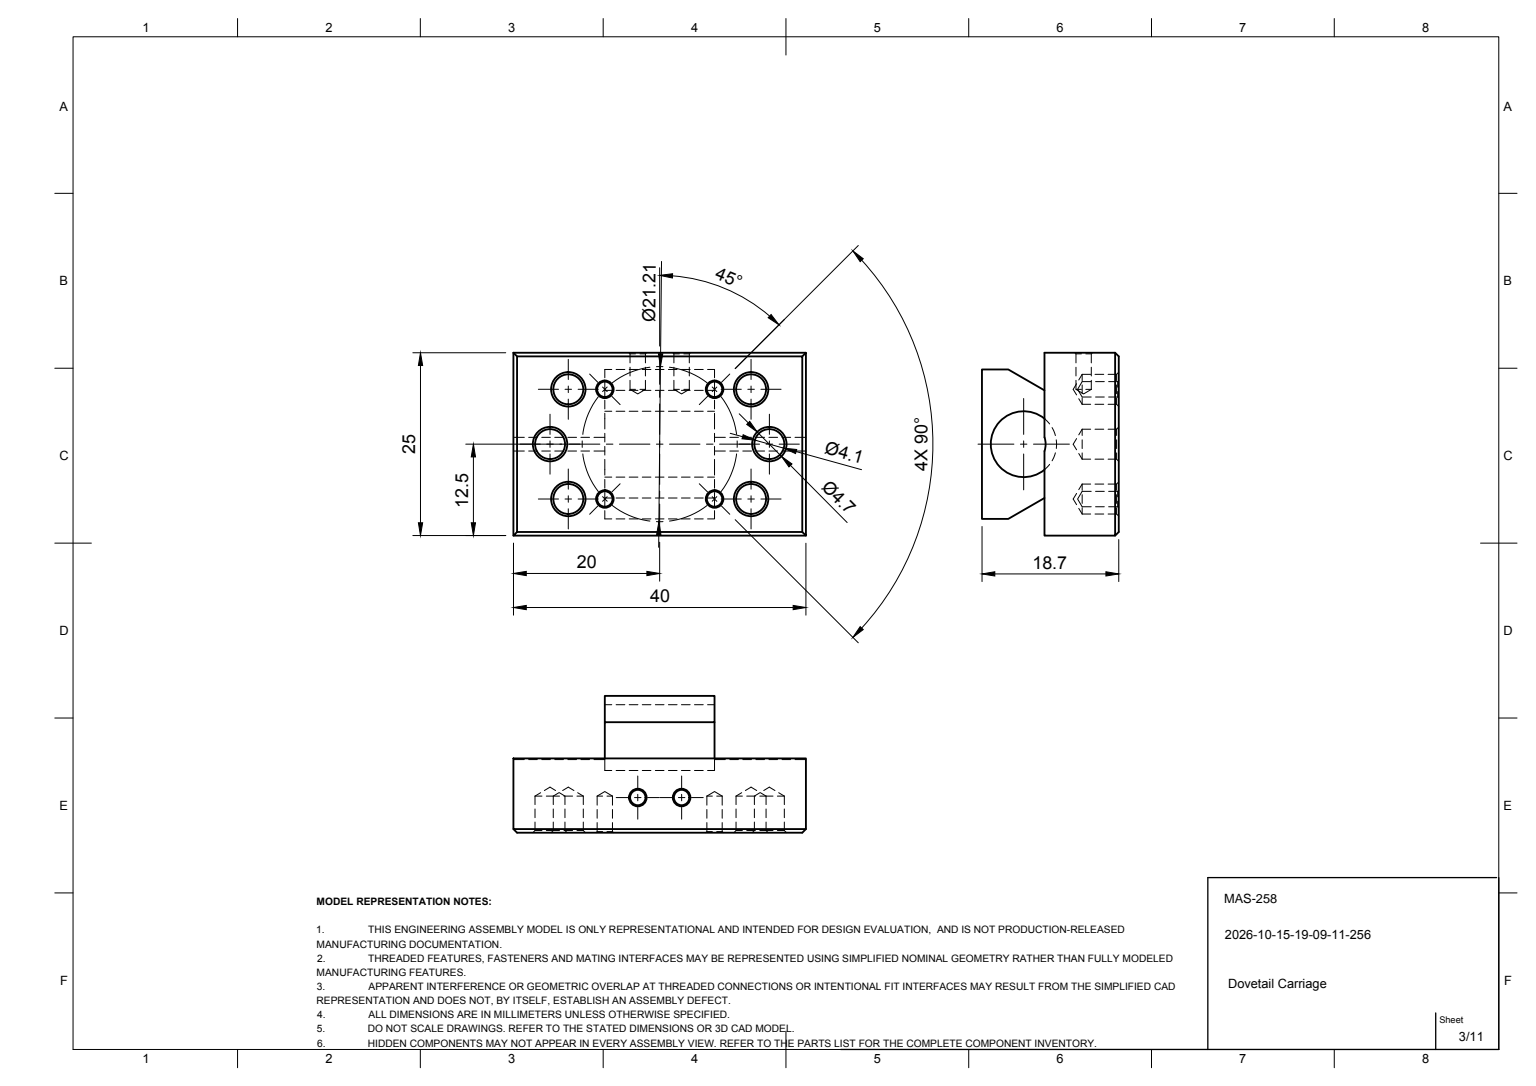
ISO-10303-21;
HEADER;
/* Generated by software containing ST-Developer
 * from STEP Tools, Inc. (www.steptools.com) 
 */

FILE_DESCRIPTION(
/* description */ (''),
/* implementation_level */ '2;1');

FILE_NAME(
/* name */ 'Dovetail Carriage.step',
/* time_stamp */ '2026-10-15T12:29:06-07:00',
/* author */ (''),
/* organization */ (''),
/* preprocessor_version */ 'ST-DEVELOPER v20.2',
/* originating_system */ 'Autodesk Translation Framework v15.15.0.0',
/* authorisation */ '');

FILE_SCHEMA (('AUTOMOTIVE_DESIGN { 1 0 10303 214 3 1 1 }'));
ENDSEC;

DATA;
#10=MECHANICAL_DESIGN_GEOMETRIC_PRESENTATION_REPRESENTATION('',(#1740),#135282);
#1714=SHAPE_REPRESENTATION_RELATIONSHIP('SRR','None',#135338,#1727);
#1727=ADVANCED_BREP_SHAPE_REPRESENTATION('',(#1753),#135270);
#1740=STYLED_ITEM('',(#135412),#1753);
#1753=MANIFOLD_SOLID_BREP('Body1',#32076);
#1769=CYLINDRICAL_SURFACE('',#32282,1.05);
#1770=CYLINDRICAL_SURFACE('',#32287,1.05);
#1771=CYLINDRICAL_SURFACE('',#32305,1.05);
#1772=CYLINDRICAL_SURFACE('',#32309,1.05);
#1773=CYLINDRICAL_SURFACE('',#32313,1.05);
#1774=CYLINDRICAL_SURFACE('',#32317,1.05);
#1775=CYLINDRICAL_SURFACE('',#32325,2.05);
#1776=CYLINDRICAL_SURFACE('',#32329,2.05);
#1777=CYLINDRICAL_SURFACE('',#32333,2.05);
#1778=CYLINDRICAL_SURFACE('',#32337,2.05);
#1779=CYLINDRICAL_SURFACE('',#32341,2.05);
#1780=CYLINDRICAL_SURFACE('',#32345,2.05);
#1781=CYLINDRICAL_SURFACE('',#32353,3.);
#1782=CYLINDRICAL_SURFACE('',#32358,3.);
#1783=CYLINDRICAL_SURFACE('',#32365,4.5);
#2020=FACE_BOUND('',#5136,.T.);
#2021=FACE_BOUND('',#5137,.T.);
#2022=FACE_BOUND('',#5145,.T.);
#2023=FACE_BOUND('',#5146,.T.);
#2024=FACE_BOUND('',#5147,.T.);
#2025=FACE_BOUND('',#5148,.T.);
#2026=FACE_BOUND('',#5149,.T.);
#2027=FACE_BOUND('',#5150,.T.);
#2028=FACE_BOUND('',#5151,.T.);
#2029=FACE_BOUND('',#5152,.T.);
#2030=FACE_BOUND('',#5153,.T.);
#2031=FACE_BOUND('',#5154,.T.);
#2250=PLANE('',#32280);
#2251=PLANE('',#32295);
#2252=PLANE('',#32356);
#2253=PLANE('',#32357);
#2254=PLANE('',#32361);
#2255=PLANE('',#32363);
#2256=PLANE('',#32370);
#2257=PLANE('',#32371);
#2258=PLANE('',#32372);
#2259=PLANE('',#32373);
#2260=PLANE('',#32374);
#2261=PLANE('',#32375);
#2262=PLANE('',#32376);
#2263=PLANE('',#32377);
#2264=PLANE('',#32378);
#2265=PLANE('',#32379);
#2266=PLANE('',#32380);
#2267=PLANE('',#32381);
#2268=PLANE('',#32382);
#2269=PLANE('',#32383);
#3376=FACE_OUTER_BOUND('',#5134,.T.);
#3377=FACE_OUTER_BOUND('',#5135,.T.);
#3378=FACE_OUTER_BOUND('',#5138,.T.);
#3379=FACE_OUTER_BOUND('',#5139,.T.);
#3380=FACE_OUTER_BOUND('',#5140,.T.);
#3381=FACE_OUTER_BOUND('',#5141,.T.);
#3382=FACE_OUTER_BOUND('',#5142,.T.);
#3383=FACE_OUTER_BOUND('',#5143,.T.);
#3384=FACE_OUTER_BOUND('',#5144,.T.);
#3385=FACE_OUTER_BOUND('',#5155,.T.);
#3386=FACE_OUTER_BOUND('',#5156,.T.);
#3387=FACE_OUTER_BOUND('',#5157,.T.);
#3388=FACE_OUTER_BOUND('',#5158,.T.);
#3389=FACE_OUTER_BOUND('',#5159,.T.);
#3390=FACE_OUTER_BOUND('',#5160,.T.);
#3391=FACE_OUTER_BOUND('',#5161,.T.);
#3392=FACE_OUTER_BOUND('',#5162,.T.);
#3393=FACE_OUTER_BOUND('',#5163,.T.);
#3394=FACE_OUTER_BOUND('',#5164,.T.);
#3395=FACE_OUTER_BOUND('',#5165,.T.);
#3396=FACE_OUTER_BOUND('',#5166,.T.);
#3397=FACE_OUTER_BOUND('',#5167,.T.);
#3398=FACE_OUTER_BOUND('',#5168,.T.);
#3399=FACE_OUTER_BOUND('',#5169,.T.);
#3400=FACE_OUTER_BOUND('',#5170,.T.);
#3401=FACE_OUTER_BOUND('',#5171,.T.);
#3402=FACE_OUTER_BOUND('',#5172,.T.);
#3403=FACE_OUTER_BOUND('',#5173,.T.);
#3404=FACE_OUTER_BOUND('',#5174,.T.);
#3405=FACE_OUTER_BOUND('',#5175,.T.);
#3406=FACE_OUTER_BOUND('',#5176,.T.);
#3407=FACE_OUTER_BOUND('',#5177,.T.);
#3408=FACE_OUTER_BOUND('',#5178,.T.);
#3409=FACE_OUTER_BOUND('',#5179,.T.);
#3410=FACE_OUTER_BOUND('',#5180,.T.);
#3411=FACE_OUTER_BOUND('',#5181,.T.);
#3412=FACE_OUTER_BOUND('',#5182,.T.);
#3413=FACE_OUTER_BOUND('',#5183,.T.);
#3414=FACE_OUTER_BOUND('',#5184,.T.);
#3415=FACE_OUTER_BOUND('',#5185,.T.);
#3416=FACE_OUTER_BOUND('',#5186,.T.);
#3417=FACE_OUTER_BOUND('',#5187,.T.);
#3418=FACE_OUTER_BOUND('',#5188,.T.);
#3419=FACE_OUTER_BOUND('',#5189,.T.);
#3420=FACE_OUTER_BOUND('',#5190,.T.);
#3421=FACE_OUTER_BOUND('',#5191,.T.);
#3422=FACE_OUTER_BOUND('',#5192,.T.);
#3423=FACE_OUTER_BOUND('',#5193,.T.);
#3424=FACE_OUTER_BOUND('',#5194,.T.);
#3425=FACE_OUTER_BOUND('',#5195,.T.);
#3426=FACE_OUTER_BOUND('',#5196,.T.);
#3427=FACE_OUTER_BOUND('',#5197,.T.);
#3428=FACE_OUTER_BOUND('',#5198,.T.);
#3429=FACE_OUTER_BOUND('',#5199,.T.);
#3430=FACE_OUTER_BOUND('',#5200,.T.);
#3431=FACE_OUTER_BOUND('',#5201,.T.);
#3432=FACE_OUTER_BOUND('',#5202,.T.);
#3433=FACE_OUTER_BOUND('',#5203,.T.);
#3434=FACE_OUTER_BOUND('',#5204,.T.);
#5134=EDGE_LOOP('',(#21120,#21121,#21122,#21123));
#5135=EDGE_LOOP('',(#21124,#21125,#21126,#21127));
#5136=EDGE_LOOP('',(#21128));
#5137=EDGE_LOOP('',(#21129));
#5138=EDGE_LOOP('',(#21130,#21131,#21132,#21133,#21134));
#5139=EDGE_LOOP('',(#21135,#21136,#21137,#21138));
#5140=EDGE_LOOP('',(#21139,#21140,#21141,#21142,#21143));
#5141=EDGE_LOOP('',(#21144,#21145,#21146,#21147));
#5142=EDGE_LOOP('',(#21148,#21149,#21150,#21151));
#5143=EDGE_LOOP('',(#21152,#21153,#21154,#21155));
#5144=EDGE_LOOP('',(#21156,#21157,#21158,#21159));
#5145=EDGE_LOOP('',(#21160));
#5146=EDGE_LOOP('',(#21161));
#5147=EDGE_LOOP('',(#21162));
#5148=EDGE_LOOP('',(#21163));
#5149=EDGE_LOOP('',(#21164));
#5150=EDGE_LOOP('',(#21165));
#5151=EDGE_LOOP('',(#21166));
#5152=EDGE_LOOP('',(#21167));
#5153=EDGE_LOOP('',(#21168));
#5154=EDGE_LOOP('',(#21169));
#5155=EDGE_LOOP('',(#21170,#21171,#21172,#21173));
#5156=EDGE_LOOP('',(#21174,#21175,#21176,#21177));
#5157=EDGE_LOOP('',(#21178,#21179,#21180,#21181));
#5158=EDGE_LOOP('',(#21182,#21183,#21184,#21185));
#5159=EDGE_LOOP('',(#21186,#21187,#21188,#21189));
#5160=EDGE_LOOP('',(#21190,#21191,#21192,#21193));
#5161=EDGE_LOOP('',(#21194,#21195,#21196,#21197));
#5162=EDGE_LOOP('',(#21198,#21199,#21200));
#5163=EDGE_LOOP('',(#21201,#21202,#21203));
#5164=EDGE_LOOP('',(#21204,#21205,#21206));
#5165=EDGE_LOOP('',(#21207,#21208,#21209));
#5166=EDGE_LOOP('',(#21210,#21211,#21212,#21213));
#5167=EDGE_LOOP('',(#21214,#21215,#21216,#21217));
#5168=EDGE_LOOP('',(#21218,#21219,#21220,#21221));
#5169=EDGE_LOOP('',(#21222,#21223,#21224,#21225));
#5170=EDGE_LOOP('',(#21226,#21227,#21228,#21229));
#5171=EDGE_LOOP('',(#21230,#21231,#21232,#21233));
#5172=EDGE_LOOP('',(#21234,#21235,#21236,#21237));
#5173=EDGE_LOOP('',(#21238,#21239,#21240,#21241));
#5174=EDGE_LOOP('',(#21242,#21243,#21244,#21245));
#5175=EDGE_LOOP('',(#21246,#21247,#21248,#21249));
#5176=EDGE_LOOP('',(#21250,#21251,#21252,#21253));
#5177=EDGE_LOOP('',(#21254,#21255,#21256,#21257));
#5178=EDGE_LOOP('',(#21258,#21259,#21260));
#5179=EDGE_LOOP('',(#21261,#21262,#21263));
#5180=EDGE_LOOP('',(#21264,#21265,#21266));
#5181=EDGE_LOOP('',(#21267,#21268,#21269));
#5182=EDGE_LOOP('',(#21270,#21271,#21272));
#5183=EDGE_LOOP('',(#21273,#21274,#21275));
#5184=EDGE_LOOP('',(#21276,#21277,#21278,#21279));
#5185=EDGE_LOOP('',(#21280,#21281,#21282,#21283,#21284,#21285));
#5186=EDGE_LOOP('',(#21286,#21287,#21288,#21289,#21290,#21291,#21292,#21293,
#21294,#21295));
#5187=EDGE_LOOP('',(#21296,#21297,#21298,#21299));
#5188=EDGE_LOOP('',(#21300,#21301,#21302,#21303));
#5189=EDGE_LOOP('',(#21304,#21305,#21306,#21307));
#5190=EDGE_LOOP('',(#21308,#21309,#21310,#21311,#21312,#21313,#21314,#21315));
#5191=EDGE_LOOP('',(#21316,#21317,#21318,#21319));
#5192=EDGE_LOOP('',(#21320,#21321,#21322,#21323));
#5193=EDGE_LOOP('',(#21324,#21325,#21326,#21327));
#5194=EDGE_LOOP('',(#21328,#21329,#21330,#21331));
#5195=EDGE_LOOP('',(#21332,#21333,#21334,#21335,#21336,#21337));
#5196=EDGE_LOOP('',(#21338,#21339,#21340,#21341,#21342,#21343,#21344,#21345,
#21346));
#5197=EDGE_LOOP('',(#21347,#21348,#21349,#21350));
#5198=EDGE_LOOP('',(#21351,#21352,#21353,#21354));
#5199=EDGE_LOOP('',(#21355,#21356,#21357,#21358));
#5200=EDGE_LOOP('',(#21359,#21360,#21361,#21362));
#5201=EDGE_LOOP('',(#21363,#21364,#21365,#21366));
#5202=EDGE_LOOP('',(#21367,#21368,#21369,#21370,#21371,#21372,#21373,#21374,
#21375));
#5203=EDGE_LOOP('',(#21376,#21377,#21378,#21379));
#5204=EDGE_LOOP('',(#21380,#21381,#21382,#21383,#21384,#21385,#21386,#21387,
#21388,#21389));
#7130=LINE('',#41202,#9967);
#7131=LINE('',#41207,#9968);
#7132=LINE('',#41209,#9969);
#7133=LINE('',#41211,#9970);
#7134=LINE('',#41212,#9971);
#7135=LINE('',#41217,#9972);
#7136=LINE('',#41224,#9973);
#7137=LINE('',#41227,#9974);
#7138=LINE('',#41233,#9975);
#7139=LINE('',#41236,#9976);
#7140=LINE('',#41241,#9977);
#7141=LINE('',#41246,#9978);
#7142=LINE('',#41248,#9979);
#7143=LINE('',#41250,#9980);
#7144=LINE('',#41251,#9981);
#7145=LINE('',#41272,#9982);
#7146=LINE('',#41277,#9983);
#7147=LINE('',#41280,#9984);
#7148=LINE('',#41285,#9985);
#7149=LINE('',#41288,#9986);
#7150=LINE('',#41293,#9987);
#7151=LINE('',#41296,#9988);
#7152=LINE('',#41300,#9989);
#7153=LINE('',#41303,#9990);
#7154=LINE('',#41306,#9991);
#7155=LINE('',#41309,#9992);
#7156=LINE('',#41313,#9993);
#7157=LINE('',#41316,#9994);
#7158=LINE('',#41321,#9995);
#7159=LINE('',#41324,#9996);
#7160=LINE('',#41329,#9997);
#7161=LINE('',#41332,#9998);
#7162=LINE('',#41337,#9999);
#7163=LINE('',#41340,#10000);
#7164=LINE('',#41345,#10001);
#7165=LINE('',#41348,#10002);
#7166=LINE('',#41353,#10003);
#7167=LINE('',#41356,#10004);
#7168=LINE('',#41360,#10005);
#7169=LINE('',#41363,#10006);
#7170=LINE('',#41366,#10007);
#7171=LINE('',#41369,#10008);
#7172=LINE('',#41372,#10009);
#7173=LINE('',#41375,#10010);
#7174=LINE('',#41379,#10011);
#7175=LINE('',#41383,#10012);
#7176=LINE('',#41387,#10013);
#7177=LINE('',#41389,#10014);
#7178=LINE('',#41390,#10015);
#7179=LINE('',#41391,#10016);
#7180=LINE('',#41394,#10017);
#7181=LINE('',#41396,#10018);
#7182=LINE('',#41398,#10019);
#7183=LINE('',#41400,#10020);
#7184=LINE('',#41402,#10021);
#7185=LINE('',#41404,#10022);
#7186=LINE('',#41406,#10023);
#7187=LINE('',#41407,#10024);
#7188=LINE('',#41411,#10025);
#7189=LINE('',#41417,#10026);
#7190=LINE('',#41420,#10027);
#7191=LINE('',#41427,#10028);
#7192=LINE('',#41432,#10029);
#7193=LINE('',#41433,#10030);
#7194=LINE('',#41434,#10031);
#7195=LINE('',#41436,#10032);
#7196=LINE('',#41437,#10033);
#7197=LINE('',#41439,#10034);
#7198=LINE('',#41442,#10035);
#7199=LINE('',#41443,#10036);
#7200=LINE('',#41446,#10037);
#7201=LINE('',#41448,#10038);
#7202=LINE('',#41450,#10039);
#7203=LINE('',#41452,#10040);
#7204=LINE('',#41454,#10041);
#7205=LINE('',#41455,#10042);
#7206=LINE('',#41458,#10043);
#7207=LINE('',#41459,#10044);
#7208=LINE('',#41462,#10045);
#7209=LINE('',#41463,#10046);
#7210=LINE('',#41466,#10047);
#7211=LINE('',#41467,#10048);
#7212=LINE('',#41470,#10049);
#7213=LINE('',#41471,#10050);
#7214=LINE('',#41474,#10051);
#7215=LINE('',#41475,#10052);
#7216=LINE('',#41477,#10053);
#9967=VECTOR('',#34378,1.125);
#9968=VECTOR('',#34383,10.);
#9969=VECTOR('',#34384,10.);
#9970=VECTOR('',#34385,10.);
#9971=VECTOR('',#34386,10.);
#9972=VECTOR('',#34391,1.05);
#9973=VECTOR('',#34400,1.125);
#9974=VECTOR('',#34403,1.05);
#9975=VECTOR('',#34410,0.524999999999993);
#9976=VECTOR('',#34413,0.524999999999993);
#9977=VECTOR('',#34418,1.125);
#9978=VECTOR('',#34423,10.);
#9979=VECTOR('',#34424,10.);
#9980=VECTOR('',#34425,10.);
#9981=VECTOR('',#34426,10.);
#9982=VECTOR('',#34447,1.05);
#9983=VECTOR('',#34454,1.125);
#9984=VECTOR('',#34457,1.05);
#9985=VECTOR('',#34464,1.125);
#9986=VECTOR('',#34467,1.05);
#9987=VECTOR('',#34474,1.125);
#9988=VECTOR('',#34477,1.05);
#9989=VECTOR('',#34482,0.525);
#9990=VECTOR('',#34485,0.525);
#9991=VECTOR('',#34488,0.525);
#9992=VECTOR('',#34491,0.525);
#9993=VECTOR('',#34496,2.2);
#9994=VECTOR('',#34499,2.05);
#9995=VECTOR('',#34506,2.2);
#9996=VECTOR('',#34509,2.05);
#9997=VECTOR('',#34516,2.2);
#9998=VECTOR('',#34519,2.05);
#9999=VECTOR('',#34526,2.2);
#10000=VECTOR('',#34529,2.05);
#10001=VECTOR('',#34536,2.2);
#10002=VECTOR('',#34539,2.05);
#10003=VECTOR('',#34546,2.2);
#10004=VECTOR('',#34549,2.05);
#10005=VECTOR('',#34554,1.025);
#10006=VECTOR('',#34557,1.025);
#10007=VECTOR('',#34560,1.025);
#10008=VECTOR('',#34563,1.025);
#10009=VECTOR('',#34566,1.025);
#10010=VECTOR('',#34569,1.025);
#10011=VECTOR('',#34572,10.);
#10012=VECTOR('',#34575,10.);
#10013=VECTOR('',#34580,10.);
#10014=VECTOR('',#34581,10.);
#10015=VECTOR('',#34582,10.);
#10016=VECTOR('',#34583,10.);
#10017=VECTOR('',#34586,10.);
#10018=VECTOR('',#34587,10.);
#10019=VECTOR('',#34588,10.);
#10020=VECTOR('',#34589,10.);
#10021=VECTOR('',#34590,10.);
#10022=VECTOR('',#34591,10.);
#10023=VECTOR('',#34592,10.);
#10024=VECTOR('',#34593,10.);
#10025=VECTOR('',#34596,10.);
#10026=VECTOR('',#34605,10.);
#10027=VECTOR('',#34608,10.);
#10028=VECTOR('',#34617,4.5);
#10029=VECTOR('',#34624,10.);
#10030=VECTOR('',#34625,10.);
#10031=VECTOR('',#34626,10.);
#10032=VECTOR('',#34629,10.);
#10033=VECTOR('',#34630,10.);
#10034=VECTOR('',#34633,10.);
#10035=VECTOR('',#34638,10.);
#10036=VECTOR('',#34639,10.);
#10037=VECTOR('',#34642,10.);
#10038=VECTOR('',#34643,10.);
#10039=VECTOR('',#34644,10.);
#10040=VECTOR('',#34645,10.);
#10041=VECTOR('',#34646,10.);
#10042=VECTOR('',#34647,10.);
#10043=VECTOR('',#34650,10.);
#10044=VECTOR('',#34651,10.);
#10045=VECTOR('',#34654,10.);
#10046=VECTOR('',#34655,10.);
#10047=VECTOR('',#34658,10.);
#10048=VECTOR('',#34659,10.);
#10049=VECTOR('',#34662,10.);
#10050=VECTOR('',#34663,10.);
#10051=VECTOR('',#34666,10.);
#10052=VECTOR('',#34667,10.);
#10053=VECTOR('',#34670,10.);
#12756=CIRCLE('',#32278,1.05);
#12757=CIRCLE('',#32279,1.2);
#12758=CIRCLE('',#32281,1.2);
#12759=CIRCLE('',#32283,1.05);
#12760=CIRCLE('',#32284,1.05);
#12761=CIRCLE('',#32286,1.05);
#12762=CIRCLE('',#32288,1.05);
#12763=CIRCLE('',#32289,1.05);
#12764=CIRCLE('',#32293,1.05);
#12765=CIRCLE('',#32294,1.2);
#12766=CIRCLE('',#32296,1.2);
#12767=CIRCLE('',#32297,1.2);
#12768=CIRCLE('',#32298,2.35);
#12769=CIRCLE('',#32299,2.35);
#12770=CIRCLE('',#32300,2.35);
#12771=CIRCLE('',#32301,2.35);
#12772=CIRCLE('',#32302,2.35);
#12773=CIRCLE('',#32303,2.35);
#12774=CIRCLE('',#32304,1.2);
#12775=CIRCLE('',#32306,1.05);
#12776=CIRCLE('',#32308,1.05);
#12777=CIRCLE('',#32310,1.05);
#12778=CIRCLE('',#32312,1.05);
#12779=CIRCLE('',#32314,1.05);
#12780=CIRCLE('',#32316,1.05);
#12781=CIRCLE('',#32318,1.05);
#12782=CIRCLE('',#32324,2.05);
#12783=CIRCLE('',#32326,2.05);
#12784=CIRCLE('',#32328,2.05);
#12785=CIRCLE('',#32330,2.05);
#12786=CIRCLE('',#32332,2.05);
#12787=CIRCLE('',#32334,2.05);
#12788=CIRCLE('',#32336,2.05);
#12789=CIRCLE('',#32338,2.05);
#12790=CIRCLE('',#32340,2.05);
#12791=CIRCLE('',#32342,2.05);
#12792=CIRCLE('',#32344,2.05);
#12793=CIRCLE('',#32346,2.05);
#12794=CIRCLE('',#32354,3.);
#12795=CIRCLE('',#32355,3.);
#12796=CIRCLE('',#32359,3.);
#12797=CIRCLE('',#32360,3.);
#12798=CIRCLE('',#32362,4.5);
#12799=CIRCLE('',#32364,4.5);
#12800=CIRCLE('',#32366,4.5);
#12801=CIRCLE('',#32367,4.5);
#12802=CIRCLE('',#32368,4.5);
#12803=CIRCLE('',#32369,4.5);
#13292=VERTEX_POINT('',#41199);
#13293=VERTEX_POINT('',#41201);
#13294=VERTEX_POINT('',#41205);
#13295=VERTEX_POINT('',#41206);
#13296=VERTEX_POINT('',#41208);
#13297=VERTEX_POINT('',#41210);
#13298=VERTEX_POINT('',#41213);
#13299=VERTEX_POINT('',#41216);
#13300=VERTEX_POINT('',#41218);
#13301=VERTEX_POINT('',#41222);
#13302=VERTEX_POINT('',#41226);
#13303=VERTEX_POINT('',#41228);
#13304=VERTEX_POINT('',#41232);
#13305=VERTEX_POINT('',#41235);
#13306=VERTEX_POINT('',#41238);
#13307=VERTEX_POINT('',#41240);
#13308=VERTEX_POINT('',#41244);
#13309=VERTEX_POINT('',#41245);
#13310=VERTEX_POINT('',#41247);
#13311=VERTEX_POINT('',#41249);
#13312=VERTEX_POINT('',#41252);
#13313=VERTEX_POINT('',#41254);
#13314=VERTEX_POINT('',#41256);
#13315=VERTEX_POINT('',#41258);
#13316=VERTEX_POINT('',#41260);
#13317=VERTEX_POINT('',#41262);
#13318=VERTEX_POINT('',#41264);
#13319=VERTEX_POINT('',#41266);
#13320=VERTEX_POINT('',#41268);
#13321=VERTEX_POINT('',#41271);
#13322=VERTEX_POINT('',#41275);
#13323=VERTEX_POINT('',#41279);
#13324=VERTEX_POINT('',#41283);
#13325=VERTEX_POINT('',#41287);
#13326=VERTEX_POINT('',#41291);
#13327=VERTEX_POINT('',#41295);
#13328=VERTEX_POINT('',#41299);
#13329=VERTEX_POINT('',#41302);
#13330=VERTEX_POINT('',#41305);
#13331=VERTEX_POINT('',#41308);
#13332=VERTEX_POINT('',#41311);
#13333=VERTEX_POINT('',#41315);
#13334=VERTEX_POINT('',#41319);
#13335=VERTEX_POINT('',#41323);
#13336=VERTEX_POINT('',#41327);
#13337=VERTEX_POINT('',#41331);
#13338=VERTEX_POINT('',#41335);
#13339=VERTEX_POINT('',#41339);
#13340=VERTEX_POINT('',#41343);
#13341=VERTEX_POINT('',#41347);
#13342=VERTEX_POINT('',#41351);
#13343=VERTEX_POINT('',#41355);
#13344=VERTEX_POINT('',#41359);
#13345=VERTEX_POINT('',#41362);
#13346=VERTEX_POINT('',#41365);
#13347=VERTEX_POINT('',#41368);
#13348=VERTEX_POINT('',#41371);
#13349=VERTEX_POINT('',#41374);
#13350=VERTEX_POINT('',#41377);
#13351=VERTEX_POINT('',#41378);
#13352=VERTEX_POINT('',#41380);
#13353=VERTEX_POINT('',#41382);
#13354=VERTEX_POINT('',#41386);
#13355=VERTEX_POINT('',#41388);
#13356=VERTEX_POINT('',#41393);
#13357=VERTEX_POINT('',#41395);
#13358=VERTEX_POINT('',#41397);
#13359=VERTEX_POINT('',#41399);
#13360=VERTEX_POINT('',#41401);
#13361=VERTEX_POINT('',#41403);
#13362=VERTEX_POINT('',#41405);
#13363=VERTEX_POINT('',#41409);
#13364=VERTEX_POINT('',#41410);
#13365=VERTEX_POINT('',#41415);
#13366=VERTEX_POINT('',#41419);
#13367=VERTEX_POINT('',#41423);
#13368=VERTEX_POINT('',#41426);
#13369=VERTEX_POINT('',#41431);
#13370=VERTEX_POINT('',#41445);
#13371=VERTEX_POINT('',#41447);
#13372=VERTEX_POINT('',#41449);
#13373=VERTEX_POINT('',#41451);
#13374=VERTEX_POINT('',#41453);
#13375=VERTEX_POINT('',#41457);
#13376=VERTEX_POINT('',#41461);
#13377=VERTEX_POINT('',#41465);
#13378=VERTEX_POINT('',#41469);
#13379=VERTEX_POINT('',#41473);
#16411=EDGE_CURVE('',#13292,#13292,#12756,.T.);
#16412=EDGE_CURVE('',#13292,#13293,#7130,.T.);
#16413=EDGE_CURVE('',#13293,#13293,#12757,.T.);
#16414=EDGE_CURVE('',#13294,#13295,#7131,.T.);
#16415=EDGE_CURVE('',#13296,#13294,#7132,.T.);
#16416=EDGE_CURVE('',#13296,#13297,#7133,.T.);
#16417=EDGE_CURVE('',#13295,#13297,#7134,.T.);
#16418=EDGE_CURVE('',#13298,#13298,#12758,.T.);
#16419=EDGE_CURVE('',#13292,#13299,#7135,.T.);
#16420=EDGE_CURVE('',#13299,#13300,#12759,.T.);
#16421=EDGE_CURVE('',#13300,#13299,#12760,.T.);
#16422=EDGE_CURVE('',#13301,#13301,#12761,.T.);
#16423=EDGE_CURVE('',#13301,#13298,#7136,.T.);
#16424=EDGE_CURVE('',#13301,#13302,#7137,.T.);
#16425=EDGE_CURVE('',#13302,#13303,#12762,.T.);
#16426=EDGE_CURVE('',#13303,#13302,#12763,.T.);
#16427=EDGE_CURVE('',#13304,#13300,#7138,.T.);
#16428=EDGE_CURVE('',#13305,#13303,#7139,.T.);
#16429=EDGE_CURVE('',#13306,#13306,#12764,.T.);
#16430=EDGE_CURVE('',#13306,#13307,#7140,.T.);
#16431=EDGE_CURVE('',#13307,#13307,#12765,.T.);
#16432=EDGE_CURVE('',#13308,#13309,#7141,.T.);
#16433=EDGE_CURVE('',#13310,#13308,#7142,.T.);
#16434=EDGE_CURVE('',#13311,#13310,#7143,.T.);
#16435=EDGE_CURVE('',#13309,#13311,#7144,.T.);
#16436=EDGE_CURVE('',#13312,#13312,#12766,.T.);
#16437=EDGE_CURVE('',#13313,#13313,#12767,.T.);
#16438=EDGE_CURVE('',#13314,#13314,#12768,.T.);
#16439=EDGE_CURVE('',#13315,#13315,#12769,.T.);
#16440=EDGE_CURVE('',#13316,#13316,#12770,.T.);
#16441=EDGE_CURVE('',#13317,#13317,#12771,.T.);
#16442=EDGE_CURVE('',#13318,#13318,#12772,.T.);
#16443=EDGE_CURVE('',#13319,#13319,#12773,.T.);
#16444=EDGE_CURVE('',#13320,#13320,#12774,.T.);
#16445=EDGE_CURVE('',#13306,#13321,#7145,.T.);
#16446=EDGE_CURVE('',#13321,#13321,#12775,.T.);
#16447=EDGE_CURVE('',#13322,#13322,#12776,.T.);
#16448=EDGE_CURVE('',#13322,#13312,#7146,.T.);
#16449=EDGE_CURVE('',#13322,#13323,#7147,.T.);
#16450=EDGE_CURVE('',#13323,#13323,#12777,.T.);
#16451=EDGE_CURVE('',#13324,#13324,#12778,.T.);
#16452=EDGE_CURVE('',#13324,#13320,#7148,.T.);
#16453=EDGE_CURVE('',#13324,#13325,#7149,.T.);
#16454=EDGE_CURVE('',#13325,#13325,#12779,.T.);
#16455=EDGE_CURVE('',#13326,#13326,#12780,.T.);
#16456=EDGE_CURVE('',#13326,#13313,#7150,.T.);
#16457=EDGE_CURVE('',#13326,#13327,#7151,.T.);
#16458=EDGE_CURVE('',#13327,#13327,#12781,.T.);
#16459=EDGE_CURVE('',#13328,#13321,#7152,.T.);
#16460=EDGE_CURVE('',#13329,#13327,#7153,.T.);
#16461=EDGE_CURVE('',#13330,#13325,#7154,.T.);
#16462=EDGE_CURVE('',#13331,#13323,#7155,.T.);
#16463=EDGE_CURVE('',#13332,#13332,#12782,.T.);
#16464=EDGE_CURVE('',#13332,#13314,#7156,.T.);
#16465=EDGE_CURVE('',#13332,#13333,#7157,.T.);
#16466=EDGE_CURVE('',#13333,#13333,#12783,.T.);
#16467=EDGE_CURVE('',#13334,#13334,#12784,.T.);
#16468=EDGE_CURVE('',#13334,#13319,#7158,.T.);
#16469=EDGE_CURVE('',#13334,#13335,#7159,.T.);
#16470=EDGE_CURVE('',#13335,#13335,#12785,.T.);
#16471=EDGE_CURVE('',#13336,#13336,#12786,.T.);
#16472=EDGE_CURVE('',#13336,#13315,#7160,.T.);
#16473=EDGE_CURVE('',#13336,#13337,#7161,.T.);
#16474=EDGE_CURVE('',#13337,#13337,#12787,.T.);
#16475=EDGE_CURVE('',#13338,#13338,#12788,.T.);
#16476=EDGE_CURVE('',#13338,#13318,#7162,.T.);
#16477=EDGE_CURVE('',#13338,#13339,#7163,.T.);
#16478=EDGE_CURVE('',#13339,#13339,#12789,.T.);
#16479=EDGE_CURVE('',#13340,#13340,#12790,.T.);
#16480=EDGE_CURVE('',#13340,#13316,#7164,.T.);
#16481=EDGE_CURVE('',#13340,#13341,#7165,.T.);
#16482=EDGE_CURVE('',#13341,#13341,#12791,.T.);
#16483=EDGE_CURVE('',#13342,#13342,#12792,.T.);
#16484=EDGE_CURVE('',#13342,#13317,#7166,.T.);
#16485=EDGE_CURVE('',#13342,#13343,#7167,.T.);
#16486=EDGE_CURVE('',#13343,#13343,#12793,.T.);
#16487=EDGE_CURVE('',#13344,#13333,#7168,.T.);
#16488=EDGE_CURVE('',#13345,#13343,#7169,.T.);
#16489=EDGE_CURVE('',#13346,#13335,#7170,.T.);
#16490=EDGE_CURVE('',#13347,#13337,#7171,.T.);
#16491=EDGE_CURVE('',#13348,#13339,#7172,.T.);
#16492=EDGE_CURVE('',#13349,#13341,#7173,.T.);
#16493=EDGE_CURVE('',#13350,#13351,#7174,.T.);
#16494=EDGE_CURVE('',#13352,#13350,#12794,.T.);
#16495=EDGE_CURVE('',#13353,#13352,#7175,.T.);
#16496=EDGE_CURVE('',#13351,#13353,#12795,.T.);
#16497=EDGE_CURVE('',#13353,#13354,#7176,.T.);
#16498=EDGE_CURVE('',#13354,#13355,#7177,.T.);
#16499=EDGE_CURVE('',#13295,#13355,#7178,.T.);
#16500=EDGE_CURVE('',#13297,#13351,#7179,.T.);
#16501=EDGE_CURVE('',#13352,#13356,#7180,.T.);
#16502=EDGE_CURVE('',#13356,#13357,#7181,.T.);
#16503=EDGE_CURVE('',#13357,#13358,#7182,.T.);
#16504=EDGE_CURVE('',#13358,#13359,#7183,.T.);
#16505=EDGE_CURVE('',#13359,#13360,#7184,.T.);
#16506=EDGE_CURVE('',#13360,#13361,#7185,.T.);
#16507=EDGE_CURVE('',#13362,#13361,#7186,.T.);
#16508=EDGE_CURVE('',#13362,#13354,#7187,.T.);
#16509=EDGE_CURVE('',#13363,#13364,#7188,.T.);
#16510=EDGE_CURVE('',#13361,#13363,#12796,.T.);
#16511=EDGE_CURVE('',#13364,#13360,#12797,.T.);
#16512=EDGE_CURVE('',#13359,#13365,#12798,.T.);
#16513=EDGE_CURVE('',#13364,#13365,#7189,.T.);
#16514=EDGE_CURVE('',#13366,#13350,#7190,.T.);
#16515=EDGE_CURVE('',#13356,#13366,#12799,.T.);
#16516=EDGE_CURVE('',#13365,#13367,#12800,.T.);
#16517=EDGE_CURVE('',#13367,#13359,#12801,.T.);
#16518=EDGE_CURVE('',#13367,#13368,#7191,.T.);
#16519=EDGE_CURVE('',#13356,#13368,#12802,.T.);
#16520=EDGE_CURVE('',#13368,#13366,#12803,.T.);
#16521=EDGE_CURVE('',#13309,#13369,#7192,.T.);
#16522=EDGE_CURVE('',#13369,#13294,#7193,.T.);
#16523=EDGE_CURVE('',#13294,#13308,#7194,.T.);
#16524=EDGE_CURVE('',#13355,#13369,#7195,.T.);
#16525=EDGE_CURVE('',#13311,#13355,#7196,.T.);
#16526=EDGE_CURVE('',#13295,#13310,#7197,.T.);
#16527=EDGE_CURVE('',#13363,#13296,#7198,.T.);
#16528=EDGE_CURVE('',#13369,#13362,#7199,.T.);
#16529=EDGE_CURVE('',#13370,#13366,#7200,.T.);
#16530=EDGE_CURVE('',#13370,#13371,#7201,.T.);
#16531=EDGE_CURVE('',#13371,#13372,#7202,.T.);
#16532=EDGE_CURVE('',#13372,#13373,#7203,.T.);
#16533=EDGE_CURVE('',#13373,#13374,#7204,.T.);
#16534=EDGE_CURVE('',#13374,#13357,#7205,.T.);
#16535=EDGE_CURVE('',#13358,#13375,#7206,.T.);
#16536=EDGE_CURVE('',#13375,#13374,#7207,.T.);
#16537=EDGE_CURVE('',#13375,#13376,#7208,.T.);
#16538=EDGE_CURVE('',#13376,#13373,#7209,.T.);
#16539=EDGE_CURVE('',#13376,#13377,#7210,.T.);
#16540=EDGE_CURVE('',#13377,#13372,#7211,.T.);
#16541=EDGE_CURVE('',#13377,#13378,#7212,.T.);
#16542=EDGE_CURVE('',#13378,#13371,#7213,.T.);
#16543=EDGE_CURVE('',#13378,#13379,#7214,.T.);
#16544=EDGE_CURVE('',#13379,#13370,#7215,.T.);
#16545=EDGE_CURVE('',#13365,#13379,#7216,.T.);
#21120=ORIENTED_EDGE('',*,*,#16411,.T.);
#21121=ORIENTED_EDGE('',*,*,#16412,.T.);
#21122=ORIENTED_EDGE('',*,*,#16413,.T.);
#21123=ORIENTED_EDGE('',*,*,#16412,.F.);
#21124=ORIENTED_EDGE('',*,*,#16414,.F.);
#21125=ORIENTED_EDGE('',*,*,#16415,.F.);
#21126=ORIENTED_EDGE('',*,*,#16416,.T.);
#21127=ORIENTED_EDGE('',*,*,#16417,.F.);
#21128=ORIENTED_EDGE('',*,*,#16418,.F.);
#21129=ORIENTED_EDGE('',*,*,#16413,.F.);
#21130=ORIENTED_EDGE('',*,*,#16411,.F.);
#21131=ORIENTED_EDGE('',*,*,#16419,.T.);
#21132=ORIENTED_EDGE('',*,*,#16420,.T.);
#21133=ORIENTED_EDGE('',*,*,#16421,.T.);
#21134=ORIENTED_EDGE('',*,*,#16419,.F.);
#21135=ORIENTED_EDGE('',*,*,#16422,.T.);
#21136=ORIENTED_EDGE('',*,*,#16423,.T.);
#21137=ORIENTED_EDGE('',*,*,#16418,.T.);
#21138=ORIENTED_EDGE('',*,*,#16423,.F.);
#21139=ORIENTED_EDGE('',*,*,#16422,.F.);
#21140=ORIENTED_EDGE('',*,*,#16424,.T.);
#21141=ORIENTED_EDGE('',*,*,#16425,.T.);
#21142=ORIENTED_EDGE('',*,*,#16426,.T.);
#21143=ORIENTED_EDGE('',*,*,#16424,.F.);
#21144=ORIENTED_EDGE('',*,*,#16427,.T.);
#21145=ORIENTED_EDGE('',*,*,#16420,.F.);
#21146=ORIENTED_EDGE('',*,*,#16421,.F.);
#21147=ORIENTED_EDGE('',*,*,#16427,.F.);
#21148=ORIENTED_EDGE('',*,*,#16428,.T.);
#21149=ORIENTED_EDGE('',*,*,#16425,.F.);
#21150=ORIENTED_EDGE('',*,*,#16426,.F.);
#21151=ORIENTED_EDGE('',*,*,#16428,.F.);
#21152=ORIENTED_EDGE('',*,*,#16429,.T.);
#21153=ORIENTED_EDGE('',*,*,#16430,.T.);
#21154=ORIENTED_EDGE('',*,*,#16431,.T.);
#21155=ORIENTED_EDGE('',*,*,#16430,.F.);
#21156=ORIENTED_EDGE('',*,*,#16432,.F.);
#21157=ORIENTED_EDGE('',*,*,#16433,.F.);
#21158=ORIENTED_EDGE('',*,*,#16434,.F.);
#21159=ORIENTED_EDGE('',*,*,#16435,.F.);
#21160=ORIENTED_EDGE('',*,*,#16436,.F.);
#21161=ORIENTED_EDGE('',*,*,#16437,.F.);
#21162=ORIENTED_EDGE('',*,*,#16438,.F.);
#21163=ORIENTED_EDGE('',*,*,#16439,.F.);
#21164=ORIENTED_EDGE('',*,*,#16440,.F.);
#21165=ORIENTED_EDGE('',*,*,#16441,.F.);
#21166=ORIENTED_EDGE('',*,*,#16442,.F.);
#21167=ORIENTED_EDGE('',*,*,#16443,.F.);
#21168=ORIENTED_EDGE('',*,*,#16444,.F.);
#21169=ORIENTED_EDGE('',*,*,#16431,.F.);
#21170=ORIENTED_EDGE('',*,*,#16429,.F.);
#21171=ORIENTED_EDGE('',*,*,#16445,.T.);
#21172=ORIENTED_EDGE('',*,*,#16446,.T.);
#21173=ORIENTED_EDGE('',*,*,#16445,.F.);
#21174=ORIENTED_EDGE('',*,*,#16447,.T.);
#21175=ORIENTED_EDGE('',*,*,#16448,.T.);
#21176=ORIENTED_EDGE('',*,*,#16436,.T.);
#21177=ORIENTED_EDGE('',*,*,#16448,.F.);
#21178=ORIENTED_EDGE('',*,*,#16447,.F.);
#21179=ORIENTED_EDGE('',*,*,#16449,.T.);
#21180=ORIENTED_EDGE('',*,*,#16450,.T.);
#21181=ORIENTED_EDGE('',*,*,#16449,.F.);
#21182=ORIENTED_EDGE('',*,*,#16451,.T.);
#21183=ORIENTED_EDGE('',*,*,#16452,.T.);
#21184=ORIENTED_EDGE('',*,*,#16444,.T.);
#21185=ORIENTED_EDGE('',*,*,#16452,.F.);
#21186=ORIENTED_EDGE('',*,*,#16451,.F.);
#21187=ORIENTED_EDGE('',*,*,#16453,.T.);
#21188=ORIENTED_EDGE('',*,*,#16454,.T.);
#21189=ORIENTED_EDGE('',*,*,#16453,.F.);
#21190=ORIENTED_EDGE('',*,*,#16455,.T.);
#21191=ORIENTED_EDGE('',*,*,#16456,.T.);
#21192=ORIENTED_EDGE('',*,*,#16437,.T.);
#21193=ORIENTED_EDGE('',*,*,#16456,.F.);
#21194=ORIENTED_EDGE('',*,*,#16455,.F.);
#21195=ORIENTED_EDGE('',*,*,#16457,.T.);
#21196=ORIENTED_EDGE('',*,*,#16458,.T.);
#21197=ORIENTED_EDGE('',*,*,#16457,.F.);
#21198=ORIENTED_EDGE('',*,*,#16459,.T.);
#21199=ORIENTED_EDGE('',*,*,#16446,.F.);
#21200=ORIENTED_EDGE('',*,*,#16459,.F.);
#21201=ORIENTED_EDGE('',*,*,#16460,.T.);
#21202=ORIENTED_EDGE('',*,*,#16458,.F.);
#21203=ORIENTED_EDGE('',*,*,#16460,.F.);
#21204=ORIENTED_EDGE('',*,*,#16461,.T.);
#21205=ORIENTED_EDGE('',*,*,#16454,.F.);
#21206=ORIENTED_EDGE('',*,*,#16461,.F.);
#21207=ORIENTED_EDGE('',*,*,#16462,.T.);
#21208=ORIENTED_EDGE('',*,*,#16450,.F.);
#21209=ORIENTED_EDGE('',*,*,#16462,.F.);
#21210=ORIENTED_EDGE('',*,*,#16463,.T.);
#21211=ORIENTED_EDGE('',*,*,#16464,.T.);
#21212=ORIENTED_EDGE('',*,*,#16438,.T.);
#21213=ORIENTED_EDGE('',*,*,#16464,.F.);
#21214=ORIENTED_EDGE('',*,*,#16463,.F.);
#21215=ORIENTED_EDGE('',*,*,#16465,.T.);
#21216=ORIENTED_EDGE('',*,*,#16466,.T.);
#21217=ORIENTED_EDGE('',*,*,#16465,.F.);
#21218=ORIENTED_EDGE('',*,*,#16467,.T.);
#21219=ORIENTED_EDGE('',*,*,#16468,.T.);
#21220=ORIENTED_EDGE('',*,*,#16443,.T.);
#21221=ORIENTED_EDGE('',*,*,#16468,.F.);
#21222=ORIENTED_EDGE('',*,*,#16467,.F.);
#21223=ORIENTED_EDGE('',*,*,#16469,.T.);
#21224=ORIENTED_EDGE('',*,*,#16470,.T.);
#21225=ORIENTED_EDGE('',*,*,#16469,.F.);
#21226=ORIENTED_EDGE('',*,*,#16471,.T.);
#21227=ORIENTED_EDGE('',*,*,#16472,.T.);
#21228=ORIENTED_EDGE('',*,*,#16439,.T.);
#21229=ORIENTED_EDGE('',*,*,#16472,.F.);
#21230=ORIENTED_EDGE('',*,*,#16471,.F.);
#21231=ORIENTED_EDGE('',*,*,#16473,.T.);
#21232=ORIENTED_EDGE('',*,*,#16474,.T.);
#21233=ORIENTED_EDGE('',*,*,#16473,.F.);
#21234=ORIENTED_EDGE('',*,*,#16475,.T.);
#21235=ORIENTED_EDGE('',*,*,#16476,.T.);
#21236=ORIENTED_EDGE('',*,*,#16442,.T.);
#21237=ORIENTED_EDGE('',*,*,#16476,.F.);
#21238=ORIENTED_EDGE('',*,*,#16475,.F.);
#21239=ORIENTED_EDGE('',*,*,#16477,.T.);
#21240=ORIENTED_EDGE('',*,*,#16478,.T.);
#21241=ORIENTED_EDGE('',*,*,#16477,.F.);
#21242=ORIENTED_EDGE('',*,*,#16479,.T.);
#21243=ORIENTED_EDGE('',*,*,#16480,.T.);
#21244=ORIENTED_EDGE('',*,*,#16440,.T.);
#21245=ORIENTED_EDGE('',*,*,#16480,.F.);
#21246=ORIENTED_EDGE('',*,*,#16479,.F.);
#21247=ORIENTED_EDGE('',*,*,#16481,.T.);
#21248=ORIENTED_EDGE('',*,*,#16482,.T.);
#21249=ORIENTED_EDGE('',*,*,#16481,.F.);
#21250=ORIENTED_EDGE('',*,*,#16483,.T.);
#21251=ORIENTED_EDGE('',*,*,#16484,.T.);
#21252=ORIENTED_EDGE('',*,*,#16441,.T.);
#21253=ORIENTED_EDGE('',*,*,#16484,.F.);
#21254=ORIENTED_EDGE('',*,*,#16483,.F.);
#21255=ORIENTED_EDGE('',*,*,#16485,.T.);
#21256=ORIENTED_EDGE('',*,*,#16486,.T.);
#21257=ORIENTED_EDGE('',*,*,#16485,.F.);
#21258=ORIENTED_EDGE('',*,*,#16487,.T.);
#21259=ORIENTED_EDGE('',*,*,#16466,.F.);
#21260=ORIENTED_EDGE('',*,*,#16487,.F.);
#21261=ORIENTED_EDGE('',*,*,#16488,.T.);
#21262=ORIENTED_EDGE('',*,*,#16486,.F.);
#21263=ORIENTED_EDGE('',*,*,#16488,.F.);
#21264=ORIENTED_EDGE('',*,*,#16489,.T.);
#21265=ORIENTED_EDGE('',*,*,#16470,.F.);
#21266=ORIENTED_EDGE('',*,*,#16489,.F.);
#21267=ORIENTED_EDGE('',*,*,#16490,.T.);
#21268=ORIENTED_EDGE('',*,*,#16474,.F.);
#21269=ORIENTED_EDGE('',*,*,#16490,.F.);
#21270=ORIENTED_EDGE('',*,*,#16491,.T.);
#21271=ORIENTED_EDGE('',*,*,#16478,.F.);
#21272=ORIENTED_EDGE('',*,*,#16491,.F.);
#21273=ORIENTED_EDGE('',*,*,#16492,.T.);
#21274=ORIENTED_EDGE('',*,*,#16482,.F.);
#21275=ORIENTED_EDGE('',*,*,#16492,.F.);
#21276=ORIENTED_EDGE('',*,*,#16493,.F.);
#21277=ORIENTED_EDGE('',*,*,#16494,.F.);
#21278=ORIENTED_EDGE('',*,*,#16495,.F.);
#21279=ORIENTED_EDGE('',*,*,#16496,.F.);
#21280=ORIENTED_EDGE('',*,*,#16496,.T.);
#21281=ORIENTED_EDGE('',*,*,#16497,.T.);
#21282=ORIENTED_EDGE('',*,*,#16498,.T.);
#21283=ORIENTED_EDGE('',*,*,#16499,.F.);
#21284=ORIENTED_EDGE('',*,*,#16417,.T.);
#21285=ORIENTED_EDGE('',*,*,#16500,.T.);
#21286=ORIENTED_EDGE('',*,*,#16495,.T.);
#21287=ORIENTED_EDGE('',*,*,#16501,.T.);
#21288=ORIENTED_EDGE('',*,*,#16502,.T.);
#21289=ORIENTED_EDGE('',*,*,#16503,.T.);
#21290=ORIENTED_EDGE('',*,*,#16504,.T.);
#21291=ORIENTED_EDGE('',*,*,#16505,.T.);
#21292=ORIENTED_EDGE('',*,*,#16506,.T.);
#21293=ORIENTED_EDGE('',*,*,#16507,.F.);
#21294=ORIENTED_EDGE('',*,*,#16508,.T.);
#21295=ORIENTED_EDGE('',*,*,#16497,.F.);
#21296=ORIENTED_EDGE('',*,*,#16509,.F.);
#21297=ORIENTED_EDGE('',*,*,#16510,.F.);
#21298=ORIENTED_EDGE('',*,*,#16506,.F.);
#21299=ORIENTED_EDGE('',*,*,#16511,.F.);
#21300=ORIENTED_EDGE('',*,*,#16511,.T.);
#21301=ORIENTED_EDGE('',*,*,#16505,.F.);
#21302=ORIENTED_EDGE('',*,*,#16512,.T.);
#21303=ORIENTED_EDGE('',*,*,#16513,.F.);
#21304=ORIENTED_EDGE('',*,*,#16494,.T.);
#21305=ORIENTED_EDGE('',*,*,#16514,.F.);
#21306=ORIENTED_EDGE('',*,*,#16515,.F.);
#21307=ORIENTED_EDGE('',*,*,#16501,.F.);
#21308=ORIENTED_EDGE('',*,*,#16516,.F.);
#21309=ORIENTED_EDGE('',*,*,#16512,.F.);
#21310=ORIENTED_EDGE('',*,*,#16517,.F.);
#21311=ORIENTED_EDGE('',*,*,#16518,.T.);
#21312=ORIENTED_EDGE('',*,*,#16519,.F.);
#21313=ORIENTED_EDGE('',*,*,#16515,.T.);
#21314=ORIENTED_EDGE('',*,*,#16520,.F.);
#21315=ORIENTED_EDGE('',*,*,#16518,.F.);
#21316=ORIENTED_EDGE('',*,*,#16432,.T.);
#21317=ORIENTED_EDGE('',*,*,#16521,.T.);
#21318=ORIENTED_EDGE('',*,*,#16522,.T.);
#21319=ORIENTED_EDGE('',*,*,#16523,.T.);
#21320=ORIENTED_EDGE('',*,*,#16524,.T.);
#21321=ORIENTED_EDGE('',*,*,#16521,.F.);
#21322=ORIENTED_EDGE('',*,*,#16435,.T.);
#21323=ORIENTED_EDGE('',*,*,#16525,.T.);
#21324=ORIENTED_EDGE('',*,*,#16499,.T.);
#21325=ORIENTED_EDGE('',*,*,#16525,.F.);
#21326=ORIENTED_EDGE('',*,*,#16434,.T.);
#21327=ORIENTED_EDGE('',*,*,#16526,.F.);
#21328=ORIENTED_EDGE('',*,*,#16433,.T.);
#21329=ORIENTED_EDGE('',*,*,#16523,.F.);
#21330=ORIENTED_EDGE('',*,*,#16414,.T.);
#21331=ORIENTED_EDGE('',*,*,#16526,.T.);
#21332=ORIENTED_EDGE('',*,*,#16510,.T.);
#21333=ORIENTED_EDGE('',*,*,#16527,.T.);
#21334=ORIENTED_EDGE('',*,*,#16415,.T.);
#21335=ORIENTED_EDGE('',*,*,#16522,.F.);
#21336=ORIENTED_EDGE('',*,*,#16528,.T.);
#21337=ORIENTED_EDGE('',*,*,#16507,.T.);
#21338=ORIENTED_EDGE('',*,*,#16519,.T.);
#21339=ORIENTED_EDGE('',*,*,#16520,.T.);
#21340=ORIENTED_EDGE('',*,*,#16529,.F.);
#21341=ORIENTED_EDGE('',*,*,#16530,.T.);
#21342=ORIENTED_EDGE('',*,*,#16531,.T.);
#21343=ORIENTED_EDGE('',*,*,#16532,.T.);
#21344=ORIENTED_EDGE('',*,*,#16533,.T.);
#21345=ORIENTED_EDGE('',*,*,#16534,.T.);
#21346=ORIENTED_EDGE('',*,*,#16502,.F.);
#21347=ORIENTED_EDGE('',*,*,#16535,.F.);
#21348=ORIENTED_EDGE('',*,*,#16503,.F.);
#21349=ORIENTED_EDGE('',*,*,#16534,.F.);
#21350=ORIENTED_EDGE('',*,*,#16536,.F.);
#21351=ORIENTED_EDGE('',*,*,#16537,.F.);
#21352=ORIENTED_EDGE('',*,*,#16536,.T.);
#21353=ORIENTED_EDGE('',*,*,#16533,.F.);
#21354=ORIENTED_EDGE('',*,*,#16538,.F.);
#21355=ORIENTED_EDGE('',*,*,#16539,.F.);
#21356=ORIENTED_EDGE('',*,*,#16538,.T.);
#21357=ORIENTED_EDGE('',*,*,#16532,.F.);
#21358=ORIENTED_EDGE('',*,*,#16540,.F.);
#21359=ORIENTED_EDGE('',*,*,#16541,.F.);
#21360=ORIENTED_EDGE('',*,*,#16540,.T.);
#21361=ORIENTED_EDGE('',*,*,#16531,.F.);
#21362=ORIENTED_EDGE('',*,*,#16542,.F.);
#21363=ORIENTED_EDGE('',*,*,#16543,.F.);
#21364=ORIENTED_EDGE('',*,*,#16542,.T.);
#21365=ORIENTED_EDGE('',*,*,#16530,.F.);
#21366=ORIENTED_EDGE('',*,*,#16544,.F.);
#21367=ORIENTED_EDGE('',*,*,#16516,.T.);
#21368=ORIENTED_EDGE('',*,*,#16517,.T.);
#21369=ORIENTED_EDGE('',*,*,#16504,.F.);
#21370=ORIENTED_EDGE('',*,*,#16535,.T.);
#21371=ORIENTED_EDGE('',*,*,#16537,.T.);
#21372=ORIENTED_EDGE('',*,*,#16539,.T.);
#21373=ORIENTED_EDGE('',*,*,#16541,.T.);
#21374=ORIENTED_EDGE('',*,*,#16543,.T.);
#21375=ORIENTED_EDGE('',*,*,#16545,.F.);
#21376=ORIENTED_EDGE('',*,*,#16524,.F.);
#21377=ORIENTED_EDGE('',*,*,#16498,.F.);
#21378=ORIENTED_EDGE('',*,*,#16508,.F.);
#21379=ORIENTED_EDGE('',*,*,#16528,.F.);
#21380=ORIENTED_EDGE('',*,*,#16493,.T.);
#21381=ORIENTED_EDGE('',*,*,#16500,.F.);
#21382=ORIENTED_EDGE('',*,*,#16416,.F.);
#21383=ORIENTED_EDGE('',*,*,#16527,.F.);
#21384=ORIENTED_EDGE('',*,*,#16509,.T.);
#21385=ORIENTED_EDGE('',*,*,#16513,.T.);
#21386=ORIENTED_EDGE('',*,*,#16545,.T.);
#21387=ORIENTED_EDGE('',*,*,#16544,.T.);
#21388=ORIENTED_EDGE('',*,*,#16529,.T.);
#21389=ORIENTED_EDGE('',*,*,#16514,.T.);
#30258=CONICAL_SURFACE('',#32277,1.125,0.785398163397456);
#30259=CONICAL_SURFACE('',#32285,1.125,0.785398163397456);
#30260=CONICAL_SURFACE('',#32290,0.524999999999993,1.02974425867665);
#30261=CONICAL_SURFACE('',#32291,0.524999999999993,1.02974425867665);
#30262=CONICAL_SURFACE('',#32292,1.125,0.785398163397445);
#30263=CONICAL_SURFACE('',#32307,1.125,0.785398163397445);
#30264=CONICAL_SURFACE('',#32311,1.125,0.785398163397445);
#30265=CONICAL_SURFACE('',#32315,1.125,0.785398163397445);
#30266=CONICAL_SURFACE('',#32319,0.525,1.02974425867665);
#30267=CONICAL_SURFACE('',#32320,0.525,1.02974425867665);
#30268=CONICAL_SURFACE('',#32321,0.525,1.02974425867665);
#30269=CONICAL_SURFACE('',#32322,0.525,1.02974425867665);
#30270=CONICAL_SURFACE('',#32323,2.2,0.785398163397451);
#30271=CONICAL_SURFACE('',#32327,2.2,0.785398163397452);
#30272=CONICAL_SURFACE('',#32331,2.2,0.785398163397452);
#30273=CONICAL_SURFACE('',#32335,2.2,0.785398163397452);
#30274=CONICAL_SURFACE('',#32339,2.2,0.785398163397452);
#30275=CONICAL_SURFACE('',#32343,2.2,0.785398163397451);
#30276=CONICAL_SURFACE('',#32347,1.025,1.02974425867666);
#30277=CONICAL_SURFACE('',#32348,1.025,1.02974425867666);
#30278=CONICAL_SURFACE('',#32349,1.025,1.02974425867666);
#30279=CONICAL_SURFACE('',#32350,1.025,1.02974425867666);
#30280=CONICAL_SURFACE('',#32351,1.025,1.02974425867666);
#30281=CONICAL_SURFACE('',#32352,1.025,1.02974425867666);
#30351=ADVANCED_FACE('',(#3376),#30258,.F.);
#30352=ADVANCED_FACE('',(#3377,#2020,#2021),#2250,.T.);
#30353=ADVANCED_FACE('',(#3378),#1769,.F.);
#30354=ADVANCED_FACE('',(#3379),#30259,.F.);
#30355=ADVANCED_FACE('',(#3380),#1770,.F.);
#30356=ADVANCED_FACE('',(#3381),#30260,.F.);
#30357=ADVANCED_FACE('',(#3382),#30261,.F.);
#30358=ADVANCED_FACE('',(#3383),#30262,.F.);
#30359=ADVANCED_FACE('',(#3384,#2022,#2023,#2024,#2025,#2026,#2027,#2028,
#2029,#2030,#2031),#2251,.T.);
#30360=ADVANCED_FACE('',(#3385),#1771,.F.);
#30361=ADVANCED_FACE('',(#3386),#30263,.F.);
#30362=ADVANCED_FACE('',(#3387),#1772,.F.);
#30363=ADVANCED_FACE('',(#3388),#30264,.F.);
#30364=ADVANCED_FACE('',(#3389),#1773,.F.);
#30365=ADVANCED_FACE('',(#3390),#30265,.F.);
#30366=ADVANCED_FACE('',(#3391),#1774,.F.);
#30367=ADVANCED_FACE('',(#3392),#30266,.F.);
#30368=ADVANCED_FACE('',(#3393),#30267,.F.);
#30369=ADVANCED_FACE('',(#3394),#30268,.F.);
#30370=ADVANCED_FACE('',(#3395),#30269,.F.);
#30371=ADVANCED_FACE('',(#3396),#30270,.F.);
#30372=ADVANCED_FACE('',(#3397),#1775,.F.);
#30373=ADVANCED_FACE('',(#3398),#30271,.F.);
#30374=ADVANCED_FACE('',(#3399),#1776,.F.);
#30375=ADVANCED_FACE('',(#3400),#30272,.F.);
#30376=ADVANCED_FACE('',(#3401),#1777,.F.);
#30377=ADVANCED_FACE('',(#3402),#30273,.F.);
#30378=ADVANCED_FACE('',(#3403),#1778,.F.);
#30379=ADVANCED_FACE('',(#3404),#30274,.F.);
#30380=ADVANCED_FACE('',(#3405),#1779,.F.);
#30381=ADVANCED_FACE('',(#3406),#30275,.F.);
#30382=ADVANCED_FACE('',(#3407),#1780,.F.);
#30383=ADVANCED_FACE('',(#3408),#30276,.F.);
#30384=ADVANCED_FACE('',(#3409),#30277,.F.);
#30385=ADVANCED_FACE('',(#3410),#30278,.F.);
#30386=ADVANCED_FACE('',(#3411),#30279,.F.);
#30387=ADVANCED_FACE('',(#3412),#30280,.F.);
#30388=ADVANCED_FACE('',(#3413),#30281,.F.);
#30389=ADVANCED_FACE('',(#3414),#1781,.F.);
#30390=ADVANCED_FACE('',(#3415),#2252,.T.);
#30391=ADVANCED_FACE('',(#3416),#2253,.T.);
#30392=ADVANCED_FACE('',(#3417),#1782,.F.);
#30393=ADVANCED_FACE('',(#3418),#2254,.T.);
#30394=ADVANCED_FACE('',(#3419),#2255,.F.);
#30395=ADVANCED_FACE('',(#3420),#1783,.F.);
#30396=ADVANCED_FACE('',(#3421),#2256,.T.);
#30397=ADVANCED_FACE('',(#3422),#2257,.T.);
#30398=ADVANCED_FACE('',(#3423),#2258,.T.);
#30399=ADVANCED_FACE('',(#3424),#2259,.T.);
#30400=ADVANCED_FACE('',(#3425),#2260,.F.);
#30401=ADVANCED_FACE('',(#3426),#2261,.T.);
#30402=ADVANCED_FACE('',(#3427),#2262,.T.);
#30403=ADVANCED_FACE('',(#3428),#2263,.T.);
#30404=ADVANCED_FACE('',(#3429),#2264,.T.);
#30405=ADVANCED_FACE('',(#3430),#2265,.T.);
#30406=ADVANCED_FACE('',(#3431),#2266,.T.);
#30407=ADVANCED_FACE('',(#3432),#2267,.F.);
#30408=ADVANCED_FACE('',(#3433),#2268,.T.);
#30409=ADVANCED_FACE('',(#3434),#2269,.T.);
#32076=CLOSED_SHELL('',(#30351,#30352,#30353,#30354,#30355,#30356,#30357,
#30358,#30359,#30360,#30361,#30362,#30363,#30364,#30365,#30366,#30367,#30368,
#30369,#30370,#30371,#30372,#30373,#30374,#30375,#30376,#30377,#30378,#30379,
#30380,#30381,#30382,#30383,#30384,#30385,#30386,#30387,#30388,#30389,#30390,
#30391,#30392,#30393,#30394,#30395,#30396,#30397,#30398,#30399,#30400,#30401,
#30402,#30403,#30404,#30405,#30406,#30407,#30408,#30409));
#32276=AXIS2_PLACEMENT_3D('',#41197,#34372,#34373);
#32277=AXIS2_PLACEMENT_3D('',#41198,#34374,#34375);
#32278=AXIS2_PLACEMENT_3D('',#41200,#34376,#34377);
#32279=AXIS2_PLACEMENT_3D('',#41203,#34379,#34380);
#32280=AXIS2_PLACEMENT_3D('',#41204,#34381,#34382);
#32281=AXIS2_PLACEMENT_3D('',#41214,#34387,#34388);
#32282=AXIS2_PLACEMENT_3D('',#41215,#34389,#34390);
#32283=AXIS2_PLACEMENT_3D('',#41219,#34392,#34393);
#32284=AXIS2_PLACEMENT_3D('',#41220,#34394,#34395);
#32285=AXIS2_PLACEMENT_3D('',#41221,#34396,#34397);
#32286=AXIS2_PLACEMENT_3D('',#41223,#34398,#34399);
#32287=AXIS2_PLACEMENT_3D('',#41225,#34401,#34402);
#32288=AXIS2_PLACEMENT_3D('',#41229,#34404,#34405);
#32289=AXIS2_PLACEMENT_3D('',#41230,#34406,#34407);
#32290=AXIS2_PLACEMENT_3D('',#41231,#34408,#34409);
#32291=AXIS2_PLACEMENT_3D('',#41234,#34411,#34412);
#32292=AXIS2_PLACEMENT_3D('',#41237,#34414,#34415);
#32293=AXIS2_PLACEMENT_3D('',#41239,#34416,#34417);
#32294=AXIS2_PLACEMENT_3D('',#41242,#34419,#34420);
#32295=AXIS2_PLACEMENT_3D('',#41243,#34421,#34422);
#32296=AXIS2_PLACEMENT_3D('',#41253,#34427,#34428);
#32297=AXIS2_PLACEMENT_3D('',#41255,#34429,#34430);
#32298=AXIS2_PLACEMENT_3D('',#41257,#34431,#34432);
#32299=AXIS2_PLACEMENT_3D('',#41259,#34433,#34434);
#32300=AXIS2_PLACEMENT_3D('',#41261,#34435,#34436);
#32301=AXIS2_PLACEMENT_3D('',#41263,#34437,#34438);
#32302=AXIS2_PLACEMENT_3D('',#41265,#34439,#34440);
#32303=AXIS2_PLACEMENT_3D('',#41267,#34441,#34442);
#32304=AXIS2_PLACEMENT_3D('',#41269,#34443,#34444);
#32305=AXIS2_PLACEMENT_3D('',#41270,#34445,#34446);
#32306=AXIS2_PLACEMENT_3D('',#41273,#34448,#34449);
#32307=AXIS2_PLACEMENT_3D('',#41274,#34450,#34451);
#32308=AXIS2_PLACEMENT_3D('',#41276,#34452,#34453);
#32309=AXIS2_PLACEMENT_3D('',#41278,#34455,#34456);
#32310=AXIS2_PLACEMENT_3D('',#41281,#34458,#34459);
#32311=AXIS2_PLACEMENT_3D('',#41282,#34460,#34461);
#32312=AXIS2_PLACEMENT_3D('',#41284,#34462,#34463);
#32313=AXIS2_PLACEMENT_3D('',#41286,#34465,#34466);
#32314=AXIS2_PLACEMENT_3D('',#41289,#34468,#34469);
#32315=AXIS2_PLACEMENT_3D('',#41290,#34470,#34471);
#32316=AXIS2_PLACEMENT_3D('',#41292,#34472,#34473);
#32317=AXIS2_PLACEMENT_3D('',#41294,#34475,#34476);
#32318=AXIS2_PLACEMENT_3D('',#41297,#34478,#34479);
#32319=AXIS2_PLACEMENT_3D('',#41298,#34480,#34481);
#32320=AXIS2_PLACEMENT_3D('',#41301,#34483,#34484);
#32321=AXIS2_PLACEMENT_3D('',#41304,#34486,#34487);
#32322=AXIS2_PLACEMENT_3D('',#41307,#34489,#34490);
#32323=AXIS2_PLACEMENT_3D('',#41310,#34492,#34493);
#32324=AXIS2_PLACEMENT_3D('',#41312,#34494,#34495);
#32325=AXIS2_PLACEMENT_3D('',#41314,#34497,#34498);
#32326=AXIS2_PLACEMENT_3D('',#41317,#34500,#34501);
#32327=AXIS2_PLACEMENT_3D('',#41318,#34502,#34503);
#32328=AXIS2_PLACEMENT_3D('',#41320,#34504,#34505);
#32329=AXIS2_PLACEMENT_3D('',#41322,#34507,#34508);
#32330=AXIS2_PLACEMENT_3D('',#41325,#34510,#34511);
#32331=AXIS2_PLACEMENT_3D('',#41326,#34512,#34513);
#32332=AXIS2_PLACEMENT_3D('',#41328,#34514,#34515);
#32333=AXIS2_PLACEMENT_3D('',#41330,#34517,#34518);
#32334=AXIS2_PLACEMENT_3D('',#41333,#34520,#34521);
#32335=AXIS2_PLACEMENT_3D('',#41334,#34522,#34523);
#32336=AXIS2_PLACEMENT_3D('',#41336,#34524,#34525);
#32337=AXIS2_PLACEMENT_3D('',#41338,#34527,#34528);
#32338=AXIS2_PLACEMENT_3D('',#41341,#34530,#34531);
#32339=AXIS2_PLACEMENT_3D('',#41342,#34532,#34533);
#32340=AXIS2_PLACEMENT_3D('',#41344,#34534,#34535);
#32341=AXIS2_PLACEMENT_3D('',#41346,#34537,#34538);
#32342=AXIS2_PLACEMENT_3D('',#41349,#34540,#34541);
#32343=AXIS2_PLACEMENT_3D('',#41350,#34542,#34543);
#32344=AXIS2_PLACEMENT_3D('',#41352,#34544,#34545);
#32345=AXIS2_PLACEMENT_3D('',#41354,#34547,#34548);
#32346=AXIS2_PLACEMENT_3D('',#41357,#34550,#34551);
#32347=AXIS2_PLACEMENT_3D('',#41358,#34552,#34553);
#32348=AXIS2_PLACEMENT_3D('',#41361,#34555,#34556);
#32349=AXIS2_PLACEMENT_3D('',#41364,#34558,#34559);
#32350=AXIS2_PLACEMENT_3D('',#41367,#34561,#34562);
#32351=AXIS2_PLACEMENT_3D('',#41370,#34564,#34565);
#32352=AXIS2_PLACEMENT_3D('',#41373,#34567,#34568);
#32353=AXIS2_PLACEMENT_3D('',#41376,#34570,#34571);
#32354=AXIS2_PLACEMENT_3D('',#41381,#34573,#34574);
#32355=AXIS2_PLACEMENT_3D('',#41384,#34576,#34577);
#32356=AXIS2_PLACEMENT_3D('',#41385,#34578,#34579);
#32357=AXIS2_PLACEMENT_3D('',#41392,#34584,#34585);
#32358=AXIS2_PLACEMENT_3D('',#41408,#34594,#34595);
#32359=AXIS2_PLACEMENT_3D('',#41412,#34597,#34598);
#32360=AXIS2_PLACEMENT_3D('',#41413,#34599,#34600);
#32361=AXIS2_PLACEMENT_3D('',#41414,#34601,#34602);
#32362=AXIS2_PLACEMENT_3D('',#41416,#34603,#34604);
#32363=AXIS2_PLACEMENT_3D('',#41418,#34606,#34607);
#32364=AXIS2_PLACEMENT_3D('',#41421,#34609,#34610);
#32365=AXIS2_PLACEMENT_3D('',#41422,#34611,#34612);
#32366=AXIS2_PLACEMENT_3D('',#41424,#34613,#34614);
#32367=AXIS2_PLACEMENT_3D('',#41425,#34615,#34616);
#32368=AXIS2_PLACEMENT_3D('',#41428,#34618,#34619);
#32369=AXIS2_PLACEMENT_3D('',#41429,#34620,#34621);
#32370=AXIS2_PLACEMENT_3D('',#41430,#34622,#34623);
#32371=AXIS2_PLACEMENT_3D('',#41435,#34627,#34628);
#32372=AXIS2_PLACEMENT_3D('',#41438,#34631,#34632);
#32373=AXIS2_PLACEMENT_3D('',#41440,#34634,#34635);
#32374=AXIS2_PLACEMENT_3D('',#41441,#34636,#34637);
#32375=AXIS2_PLACEMENT_3D('',#41444,#34640,#34641);
#32376=AXIS2_PLACEMENT_3D('',#41456,#34648,#34649);
#32377=AXIS2_PLACEMENT_3D('',#41460,#34652,#34653);
#32378=AXIS2_PLACEMENT_3D('',#41464,#34656,#34657);
#32379=AXIS2_PLACEMENT_3D('',#41468,#34660,#34661);
#32380=AXIS2_PLACEMENT_3D('',#41472,#34664,#34665);
#32381=AXIS2_PLACEMENT_3D('',#41476,#34668,#34669);
#32382=AXIS2_PLACEMENT_3D('',#41478,#34671,#34672);
#32383=AXIS2_PLACEMENT_3D('',#41479,#34673,#34674);
#34372=DIRECTION('axis',(0.,0.,1.));
#34373=DIRECTION('refdir',(1.,0.,0.));
#34374=DIRECTION('center_axis',(1.,0.,0.));
#34375=DIRECTION('ref_axis',(0.,0.,-1.));
#34376=DIRECTION('center_axis',(-1.,0.,0.));
#34377=DIRECTION('ref_axis',(0.,0.,-1.));
#34378=DIRECTION('',(0.707106781186542,-8.659560562355E-17,0.707106781186553));
#34379=DIRECTION('center_axis',(1.,0.,0.));
#34380=DIRECTION('ref_axis',(0.,0.,-1.));
#34381=DIRECTION('center_axis',(1.,0.,0.));
#34382=DIRECTION('ref_axis',(0.,0.,-1.));
#34383=DIRECTION('',(0.,1.,0.));
#34384=DIRECTION('',(0.,0.,1.));
#34385=DIRECTION('',(0.,1.,0.));
#34386=DIRECTION('',(0.,0.,-1.));
#34387=DIRECTION('center_axis',(1.,0.,0.));
#34388=DIRECTION('ref_axis',(0.,0.,-1.));
#34389=DIRECTION('center_axis',(-1.,0.,0.));
#34390=DIRECTION('ref_axis',(0.,0.,-1.));
#34391=DIRECTION('',(-1.,0.,0.));
#34392=DIRECTION('center_axis',(-1.,0.,0.));
#34393=DIRECTION('ref_axis',(0.,0.,-1.));
#34394=DIRECTION('center_axis',(-1.,0.,0.));
#34395=DIRECTION('ref_axis',(0.,0.,-1.));
#34396=DIRECTION('center_axis',(1.,0.,0.));
#34397=DIRECTION('ref_axis',(0.,0.,-1.));
#34398=DIRECTION('center_axis',(-1.,0.,0.));
#34399=DIRECTION('ref_axis',(0.,0.,-1.));
#34400=DIRECTION('',(0.707106781186542,-8.659560562355E-17,0.707106781186553));
#34401=DIRECTION('center_axis',(-1.,0.,0.));
#34402=DIRECTION('ref_axis',(0.,0.,-1.));
#34403=DIRECTION('',(-1.,0.,0.));
#34404=DIRECTION('center_axis',(-1.,0.,0.));
#34405=DIRECTION('ref_axis',(0.,0.,-1.));
#34406=DIRECTION('center_axis',(-1.,0.,0.));
#34407=DIRECTION('ref_axis',(0.,0.,-1.));
#34408=DIRECTION('center_axis',(1.,0.,0.));
#34409=DIRECTION('ref_axis',(0.,1.,0.));
#34410=DIRECTION('',(0.515038074910058,-0.85716730070211,-1.04972719113862E-16));
#34411=DIRECTION('center_axis',(1.,0.,0.));
#34412=DIRECTION('ref_axis',(0.,1.,0.));
#34413=DIRECTION('',(0.515038074910058,-0.85716730070211,-1.04972719113862E-16));
#34414=DIRECTION('center_axis',(0.,0.,1.));
#34415=DIRECTION('ref_axis',(1.,0.,0.));
#34416=DIRECTION('center_axis',(0.,0.,-1.));
#34417=DIRECTION('ref_axis',(1.,0.,0.));
#34418=DIRECTION('',(-0.707106781186545,-8.6595605623549E-17,0.70710678118655));
#34419=DIRECTION('center_axis',(0.,0.,1.));
#34420=DIRECTION('ref_axis',(1.,0.,0.));
#34421=DIRECTION('center_axis',(0.,0.,1.));
#34422=DIRECTION('ref_axis',(1.,0.,0.));
#34423=DIRECTION('',(-1.,0.,0.));
#34424=DIRECTION('',(0.,-1.,0.));
#34425=DIRECTION('',(1.,0.,0.));
#34426=DIRECTION('',(0.,1.,0.));
#34427=DIRECTION('center_axis',(0.,0.,1.));
#34428=DIRECTION('ref_axis',(1.,0.,0.));
#34429=DIRECTION('center_axis',(0.,0.,1.));
#34430=DIRECTION('ref_axis',(1.,0.,0.));
#34431=DIRECTION('center_axis',(0.,0.,1.));
#34432=DIRECTION('ref_axis',(1.,0.,0.));
#34433=DIRECTION('center_axis',(0.,0.,1.));
#34434=DIRECTION('ref_axis',(1.,0.,0.));
#34435=DIRECTION('center_axis',(0.,0.,1.));
#34436=DIRECTION('ref_axis',(1.,0.,0.));
#34437=DIRECTION('center_axis',(0.,0.,1.));
#34438=DIRECTION('ref_axis',(1.,0.,0.));
#34439=DIRECTION('center_axis',(0.,0.,1.));
#34440=DIRECTION('ref_axis',(1.,0.,0.));
#34441=DIRECTION('center_axis',(0.,0.,1.));
#34442=DIRECTION('ref_axis',(1.,0.,0.));
#34443=DIRECTION('center_axis',(0.,0.,1.));
#34444=DIRECTION('ref_axis',(1.,0.,0.));
#34445=DIRECTION('center_axis',(0.,0.,-1.));
#34446=DIRECTION('ref_axis',(1.,0.,0.));
#34447=DIRECTION('',(0.,0.,-1.));
#34448=DIRECTION('center_axis',(0.,0.,-1.));
#34449=DIRECTION('ref_axis',(1.,0.,0.));
#34450=DIRECTION('center_axis',(0.,0.,1.));
#34451=DIRECTION('ref_axis',(1.,0.,0.));
#34452=DIRECTION('center_axis',(0.,0.,-1.));
#34453=DIRECTION('ref_axis',(1.,0.,0.));
#34454=DIRECTION('',(-0.707106781186545,-8.6595605623549E-17,0.70710678118655));
#34455=DIRECTION('center_axis',(0.,0.,-1.));
#34456=DIRECTION('ref_axis',(1.,0.,0.));
#34457=DIRECTION('',(0.,0.,-1.));
#34458=DIRECTION('center_axis',(0.,0.,-1.));
#34459=DIRECTION('ref_axis',(1.,0.,0.));
#34460=DIRECTION('center_axis',(0.,0.,1.));
#34461=DIRECTION('ref_axis',(1.,0.,0.));
#34462=DIRECTION('center_axis',(0.,0.,-1.));
#34463=DIRECTION('ref_axis',(1.,0.,0.));
#34464=DIRECTION('',(-0.707106781186545,-8.6595605623549E-17,0.70710678118655));
#34465=DIRECTION('center_axis',(0.,0.,-1.));
#34466=DIRECTION('ref_axis',(1.,0.,0.));
#34467=DIRECTION('',(0.,0.,-1.));
#34468=DIRECTION('center_axis',(0.,0.,-1.));
#34469=DIRECTION('ref_axis',(1.,0.,0.));
#34470=DIRECTION('center_axis',(0.,0.,1.));
#34471=DIRECTION('ref_axis',(1.,0.,0.));
#34472=DIRECTION('center_axis',(0.,0.,-1.));
#34473=DIRECTION('ref_axis',(1.,0.,0.));
#34474=DIRECTION('',(-0.707106781186545,-8.6595605623549E-17,0.70710678118655));
#34475=DIRECTION('center_axis',(0.,0.,-1.));
#34476=DIRECTION('ref_axis',(1.,0.,0.));
#34477=DIRECTION('',(0.,0.,-1.));
#34478=DIRECTION('center_axis',(0.,0.,-1.));
#34479=DIRECTION('ref_axis',(1.,0.,0.));
#34480=DIRECTION('center_axis',(0.,0.,1.));
#34481=DIRECTION('ref_axis',(1.,0.,0.));
#34482=DIRECTION('',(-0.85716730070211,-1.04972719113862E-16,0.515038074910058));
#34483=DIRECTION('center_axis',(0.,0.,1.));
#34484=DIRECTION('ref_axis',(1.,0.,0.));
#34485=DIRECTION('',(-0.85716730070211,-1.04972719113862E-16,0.515038074910058));
#34486=DIRECTION('center_axis',(0.,0.,1.));
#34487=DIRECTION('ref_axis',(1.,0.,0.));
#34488=DIRECTION('',(-0.85716730070211,-1.04972719113862E-16,0.515038074910058));
#34489=DIRECTION('center_axis',(0.,0.,1.));
#34490=DIRECTION('ref_axis',(1.,0.,0.));
#34491=DIRECTION('',(-0.85716730070211,-1.04972719113862E-16,0.515038074910058));
#34492=DIRECTION('center_axis',(0.,0.,1.));
#34493=DIRECTION('ref_axis',(1.,0.,0.));
#34494=DIRECTION('center_axis',(0.,0.,-1.));
#34495=DIRECTION('ref_axis',(1.,0.,0.));
#34496=DIRECTION('',(-0.707106781186549,-8.65956056235496E-17,0.707106781186546));
#34497=DIRECTION('center_axis',(0.,0.,-1.));
#34498=DIRECTION('ref_axis',(1.,0.,0.));
#34499=DIRECTION('',(0.,0.,-1.));
#34500=DIRECTION('center_axis',(0.,0.,-1.));
#34501=DIRECTION('ref_axis',(1.,0.,0.));
#34502=DIRECTION('center_axis',(0.,0.,1.));
#34503=DIRECTION('ref_axis',(1.,0.,0.));
#34504=DIRECTION('center_axis',(0.,0.,-1.));
#34505=DIRECTION('ref_axis',(1.,0.,0.));
#34506=DIRECTION('',(-0.70710678118655,-8.65956056235496E-17,0.707106781186545));
#34507=DIRECTION('center_axis',(0.,0.,-1.));
#34508=DIRECTION('ref_axis',(1.,0.,0.));
#34509=DIRECTION('',(0.,0.,-1.));
#34510=DIRECTION('center_axis',(0.,0.,-1.));
#34511=DIRECTION('ref_axis',(1.,0.,0.));
#34512=DIRECTION('center_axis',(0.,0.,1.));
#34513=DIRECTION('ref_axis',(1.,0.,0.));
#34514=DIRECTION('center_axis',(0.,0.,-1.));
#34515=DIRECTION('ref_axis',(1.,0.,0.));
#34516=DIRECTION('',(-0.70710678118655,-8.65956056235496E-17,0.707106781186545));
#34517=DIRECTION('center_axis',(0.,0.,-1.));
#34518=DIRECTION('ref_axis',(1.,0.,0.));
#34519=DIRECTION('',(0.,0.,-1.));
#34520=DIRECTION('center_axis',(0.,0.,-1.));
#34521=DIRECTION('ref_axis',(1.,0.,0.));
#34522=DIRECTION('center_axis',(0.,0.,1.));
#34523=DIRECTION('ref_axis',(1.,0.,0.));
#34524=DIRECTION('center_axis',(0.,0.,-1.));
#34525=DIRECTION('ref_axis',(1.,0.,0.));
#34526=DIRECTION('',(-0.70710678118655,-8.65956056235496E-17,0.707106781186545));
#34527=DIRECTION('center_axis',(0.,0.,-1.));
#34528=DIRECTION('ref_axis',(1.,0.,0.));
#34529=DIRECTION('',(0.,0.,-1.));
#34530=DIRECTION('center_axis',(0.,0.,-1.));
#34531=DIRECTION('ref_axis',(1.,0.,0.));
#34532=DIRECTION('center_axis',(0.,0.,1.));
#34533=DIRECTION('ref_axis',(1.,0.,0.));
#34534=DIRECTION('center_axis',(0.,0.,-1.));
#34535=DIRECTION('ref_axis',(1.,0.,0.));
#34536=DIRECTION('',(-0.70710678118655,-8.65956056235496E-17,0.707106781186545));
#34537=DIRECTION('center_axis',(0.,0.,-1.));
#34538=DIRECTION('ref_axis',(1.,0.,0.));
#34539=DIRECTION('',(0.,0.,-1.));
#34540=DIRECTION('center_axis',(0.,0.,-1.));
#34541=DIRECTION('ref_axis',(1.,0.,0.));
#34542=DIRECTION('center_axis',(0.,0.,1.));
#34543=DIRECTION('ref_axis',(1.,0.,0.));
#34544=DIRECTION('center_axis',(0.,0.,-1.));
#34545=DIRECTION('ref_axis',(1.,0.,0.));
#34546=DIRECTION('',(-0.707106781186549,-8.65956056235496E-17,0.707106781186546));
#34547=DIRECTION('center_axis',(0.,0.,-1.));
#34548=DIRECTION('ref_axis',(1.,0.,0.));
#34549=DIRECTION('',(0.,0.,-1.));
#34550=DIRECTION('center_axis',(0.,0.,-1.));
#34551=DIRECTION('ref_axis',(1.,0.,0.));
#34552=DIRECTION('center_axis',(0.,0.,1.));
#34553=DIRECTION('ref_axis',(1.,0.,0.));
#34554=DIRECTION('',(-0.857167300702115,-1.04972719113862E-16,0.515038074910049));
#34555=DIRECTION('center_axis',(0.,0.,1.));
#34556=DIRECTION('ref_axis',(1.,0.,0.));
#34557=DIRECTION('',(-0.857167300702115,-1.04972719113862E-16,0.515038074910049));
#34558=DIRECTION('center_axis',(0.,0.,1.));
#34559=DIRECTION('ref_axis',(1.,0.,0.));
#34560=DIRECTION('',(-0.857167300702115,-1.04972719113862E-16,0.515038074910049));
#34561=DIRECTION('center_axis',(0.,0.,1.));
#34562=DIRECTION('ref_axis',(1.,0.,0.));
#34563=DIRECTION('',(-0.857167300702115,-1.04972719113862E-16,0.515038074910049));
#34564=DIRECTION('center_axis',(0.,0.,1.));
#34565=DIRECTION('ref_axis',(1.,0.,0.));
#34566=DIRECTION('',(-0.857167300702115,-1.04972719113862E-16,0.515038074910049));
#34567=DIRECTION('center_axis',(0.,0.,1.));
#34568=DIRECTION('ref_axis',(1.,0.,0.));
#34569=DIRECTION('',(-0.857167300702115,-1.04972719113862E-16,0.515038074910049));
#34570=DIRECTION('center_axis',(0.,-1.,0.));
#34571=DIRECTION('ref_axis',(1.,0.,0.));
#34572=DIRECTION('',(0.,1.,0.));
#34573=DIRECTION('center_axis',(0.,1.,0.));
#34574=DIRECTION('ref_axis',(1.,0.,0.));
#34575=DIRECTION('',(0.,-1.,0.));
#34576=DIRECTION('center_axis',(0.,-1.,0.));
#34577=DIRECTION('ref_axis',(1.,0.,0.));
#34578=DIRECTION('center_axis',(0.,1.,0.));
#34579=DIRECTION('ref_axis',(0.,0.,1.));
#34580=DIRECTION('',(-1.,0.,0.));
#34581=DIRECTION('',(0.,0.,1.));
#34582=DIRECTION('',(-1.,0.,0.));
#34583=DIRECTION('',(-1.,0.,0.));
#34584=DIRECTION('center_axis',(0.,0.,-1.));
#34585=DIRECTION('ref_axis',(-1.,0.,0.));
#34586=DIRECTION('',(-1.,0.,0.));
#34587=DIRECTION('',(-1.,0.,0.));
#34588=DIRECTION('',(0.,-1.,0.));
#34589=DIRECTION('',(1.,0.,0.));
#34590=DIRECTION('',(1.,0.,0.));
#34591=DIRECTION('',(0.,-1.,0.));
#34592=DIRECTION('',(1.,0.,0.));
#34593=DIRECTION('',(0.,1.,0.));
#34594=DIRECTION('center_axis',(0.,1.,0.));
#34595=DIRECTION('ref_axis',(1.,0.,0.));
#34596=DIRECTION('',(0.,1.,0.));
#34597=DIRECTION('center_axis',(0.,1.,0.));
#34598=DIRECTION('ref_axis',(1.,0.,0.));
#34599=DIRECTION('center_axis',(0.,-1.,0.));
#34600=DIRECTION('ref_axis',(1.,0.,0.));
#34601=DIRECTION('center_axis',(0.,1.,0.));
#34602=DIRECTION('ref_axis',(1.,0.,0.));
#34603=DIRECTION('center_axis',(0.,1.,0.));
#34604=DIRECTION('ref_axis',(1.,0.,0.));
#34605=DIRECTION('',(1.,0.,0.));
#34606=DIRECTION('center_axis',(0.,1.,0.));
#34607=DIRECTION('ref_axis',(1.,0.,0.));
#34608=DIRECTION('',(-1.,0.,0.));
#34609=DIRECTION('center_axis',(0.,1.,0.));
#34610=DIRECTION('ref_axis',(1.,0.,0.));
#34611=DIRECTION('center_axis',(0.,1.,0.));
#34612=DIRECTION('ref_axis',(1.,0.,0.));
#34613=DIRECTION('center_axis',(0.,1.,0.));
#34614=DIRECTION('ref_axis',(1.,0.,0.));
#34615=DIRECTION('center_axis',(0.,1.,0.));
#34616=DIRECTION('ref_axis',(1.,0.,0.));
#34617=DIRECTION('',(0.,1.,0.));
#34618=DIRECTION('center_axis',(0.,-1.,0.));
#34619=DIRECTION('ref_axis',(1.,0.,0.));
#34620=DIRECTION('center_axis',(0.,-1.,0.));
#34621=DIRECTION('ref_axis',(1.,0.,0.));
#34622=DIRECTION('center_axis',(0.,-0.707106781186541,0.707106781186554));
#34623=DIRECTION('ref_axis',(1.,0.,0.));
#34624=DIRECTION('',(-0.577350269189622,-0.577350269189633,-0.577350269189622));
#34625=DIRECTION('',(1.,0.,0.));
#34626=DIRECTION('',(-0.577350269189622,0.577350269189633,0.577350269189622));
#34627=DIRECTION('center_axis',(-0.707106781186548,0.,0.707106781186548));
#34628=DIRECTION('ref_axis',(0.707106781186548,0.,0.707106781186548));
#34629=DIRECTION('',(0.,-1.,0.));
#34630=DIRECTION('',(-0.577350269189622,0.577350269189633,-0.577350269189622));
#34631=DIRECTION('center_axis',(0.,0.707106781186541,0.707106781186554));
#34632=DIRECTION('ref_axis',(1.,0.,0.));
#34633=DIRECTION('',(-0.577350269189622,-0.577350269189633,0.577350269189622));
#34634=DIRECTION('center_axis',(0.707106781186548,0.,0.707106781186548));
#34635=DIRECTION('ref_axis',(0.707106781186548,0.,-0.707106781186548));
#34636=DIRECTION('center_axis',(0.,1.,0.));
#34637=DIRECTION('ref_axis',(1.,0.,0.));
#34638=DIRECTION('',(1.,0.,0.));
#34639=DIRECTION('',(0.,0.,-1.));
#34640=DIRECTION('center_axis',(0.,1.,0.));
#34641=DIRECTION('ref_axis',(0.,0.,1.));
#34642=DIRECTION('',(-1.,0.,0.));
#34643=DIRECTION('',(0.5,0.,-0.866025403784439));
#34644=DIRECTION('',(0.,0.,-1.));
#34645=DIRECTION('',(-1.,0.,0.));
#34646=DIRECTION('',(0.,0.,1.));
#34647=DIRECTION('',(0.5,0.,0.866025403784439));
#34648=DIRECTION('center_axis',(-0.866025403784439,0.,0.5));
#34649=DIRECTION('ref_axis',(0.5,0.,0.866025403784439));
#34650=DIRECTION('',(-0.5,0.,-0.866025403784439));
#34651=DIRECTION('',(0.,1.,0.));
#34652=DIRECTION('center_axis',(-1.,0.,0.));
#34653=DIRECTION('ref_axis',(0.,0.,1.));
#34654=DIRECTION('',(0.,0.,-1.));
#34655=DIRECTION('',(0.,1.,0.));
#34656=DIRECTION('center_axis',(0.,0.,-1.));
#34657=DIRECTION('ref_axis',(-1.,0.,0.));
#34658=DIRECTION('',(1.,0.,0.));
#34659=DIRECTION('',(0.,1.,0.));
#34660=DIRECTION('center_axis',(1.,0.,0.));
#34661=DIRECTION('ref_axis',(0.,0.,-1.));
#34662=DIRECTION('',(0.,0.,1.));
#34663=DIRECTION('',(0.,1.,0.));
#34664=DIRECTION('center_axis',(0.866025403784439,0.,0.5));
#34665=DIRECTION('ref_axis',(0.5,0.,-0.866025403784439));
#34666=DIRECTION('',(-0.5,0.,0.866025403784439));
#34667=DIRECTION('',(0.,1.,0.));
#34668=DIRECTION('center_axis',(0.,1.,0.));
#34669=DIRECTION('ref_axis',(1.,0.,0.));
#34670=DIRECTION('',(1.,0.,0.));
#34671=DIRECTION('center_axis',(-1.,0.,0.));
#34672=DIRECTION('ref_axis',(0.,0.,1.));
#34673=DIRECTION('center_axis',(0.,0.,-1.));
#34674=DIRECTION('ref_axis',(-1.,0.,0.));
#41197=CARTESIAN_POINT('',(0.,0.,0.));
#41198=CARTESIAN_POINT('Origin',(12.425,73.,21.5));
#41199=CARTESIAN_POINT('',(12.35,73.,22.55));
#41200=CARTESIAN_POINT('Origin',(12.35,73.,21.5));
#41201=CARTESIAN_POINT('',(12.5,73.,22.7));
#41202=CARTESIAN_POINT('',(12.425,73.,22.625));
#41203=CARTESIAN_POINT('Origin',(12.5,73.,21.5));
#41204=CARTESIAN_POINT('Origin',(12.5,50.,26.3));
#41205=CARTESIAN_POINT('',(12.5,50.,25.8));
#41206=CARTESIAN_POINT('',(12.5,90.,25.8));
#41207=CARTESIAN_POINT('',(12.5,50.,25.8));
#41208=CARTESIAN_POINT('',(12.5,50.,16.15));
#41209=CARTESIAN_POINT('',(12.5,50.,16.15));
#41210=CARTESIAN_POINT('',(12.5,90.,16.15));
#41211=CARTESIAN_POINT('',(12.5,50.,16.15));
#41212=CARTESIAN_POINT('',(12.5,90.,16.15));
#41213=CARTESIAN_POINT('',(12.5,67.,22.7));
#41214=CARTESIAN_POINT('Origin',(12.5,67.,21.5));
#41215=CARTESIAN_POINT('Origin',(12.5,73.,21.5));
#41216=CARTESIAN_POINT('',(7.5,73.,22.55));
#41217=CARTESIAN_POINT('',(12.5,73.,22.55));
#41218=CARTESIAN_POINT('',(7.5,71.95,21.5));
#41219=CARTESIAN_POINT('Origin',(7.5,73.,21.5));
#41220=CARTESIAN_POINT('Origin',(7.5,73.,21.5));
#41221=CARTESIAN_POINT('Origin',(12.425,67.,21.5));
#41222=CARTESIAN_POINT('',(12.35,67.,22.55));
#41223=CARTESIAN_POINT('Origin',(12.35,67.,21.5));
#41224=CARTESIAN_POINT('',(12.425,67.,22.625));
#41225=CARTESIAN_POINT('Origin',(12.5,67.,21.5));
#41226=CARTESIAN_POINT('',(7.5,67.,22.55));
#41227=CARTESIAN_POINT('',(12.5,67.,22.55));
#41228=CARTESIAN_POINT('',(7.5,65.95,21.5));
#41229=CARTESIAN_POINT('Origin',(7.5,67.,21.5));
#41230=CARTESIAN_POINT('Origin',(7.5,67.,21.5));
#41231=CARTESIAN_POINT('Origin',(7.18454817501053,73.,21.5));
#41232=CARTESIAN_POINT('',(6.86909635002106,73.,21.5));
#41233=CARTESIAN_POINT('',(7.18454817501053,72.475,21.5));
#41234=CARTESIAN_POINT('Origin',(7.18454817501053,67.,21.5));
#41235=CARTESIAN_POINT('',(6.86909635002106,67.,21.5));
#41236=CARTESIAN_POINT('',(7.18454817501053,66.475,21.5));
#41237=CARTESIAN_POINT('Origin',(7.5,77.5,26.225));
#41238=CARTESIAN_POINT('',(6.45,77.5,26.15));
#41239=CARTESIAN_POINT('Origin',(7.5,77.5,26.15));
#41240=CARTESIAN_POINT('',(6.3,77.5,26.3));
#41241=CARTESIAN_POINT('',(6.375,77.5,26.225));
#41242=CARTESIAN_POINT('Origin',(7.5,77.5,26.3));
#41243=CARTESIAN_POINT('Origin',(-12.5,50.,26.3));
#41244=CARTESIAN_POINT('',(12.,50.5,26.3));
#41245=CARTESIAN_POINT('',(-12.,50.5,26.3));
#41246=CARTESIAN_POINT('',(-6.25,50.5,26.3));
#41247=CARTESIAN_POINT('',(12.,89.5,26.3));
#41248=CARTESIAN_POINT('',(12.,50.,26.3));
#41249=CARTESIAN_POINT('',(-12.,89.5,26.3));
#41250=CARTESIAN_POINT('',(-6.25,89.5,26.3));
#41251=CARTESIAN_POINT('',(-12.,50.,26.3));
#41252=CARTESIAN_POINT('',(-8.7,62.5,26.3));
#41253=CARTESIAN_POINT('Origin',(-7.5,62.5,26.3));
#41254=CARTESIAN_POINT('',(6.3,62.5,26.3));
#41255=CARTESIAN_POINT('Origin',(7.5,62.5,26.3));
#41256=CARTESIAN_POINT('',(-2.35,85.,26.3));
#41257=CARTESIAN_POINT('Origin',(0.,85.,26.3));
#41258=CARTESIAN_POINT('',(5.15,57.5,26.3));
#41259=CARTESIAN_POINT('Origin',(7.5,57.5,26.3));
#41260=CARTESIAN_POINT('',(-9.85,57.5,26.3));
#41261=CARTESIAN_POINT('Origin',(-7.5,57.5,26.3));
#41262=CARTESIAN_POINT('',(-2.35,55.,26.3));
#41263=CARTESIAN_POINT('Origin',(0.,55.,26.3));
#41264=CARTESIAN_POINT('',(-9.85,82.5,26.3));
#41265=CARTESIAN_POINT('Origin',(-7.5,82.5,26.3));
#41266=CARTESIAN_POINT('',(5.15,82.5,26.3));
#41267=CARTESIAN_POINT('Origin',(7.5,82.5,26.3));
#41268=CARTESIAN_POINT('',(-8.7,77.5,26.3));
#41269=CARTESIAN_POINT('Origin',(-7.5,77.5,26.3));
#41270=CARTESIAN_POINT('Origin',(7.5,77.5,26.3));
#41271=CARTESIAN_POINT('',(6.45,77.5,21.3));
#41272=CARTESIAN_POINT('',(6.45,77.5,26.3));
#41273=CARTESIAN_POINT('Origin',(7.5,77.5,21.3));
#41274=CARTESIAN_POINT('Origin',(-7.5,62.5,26.225));
#41275=CARTESIAN_POINT('',(-8.55,62.5,26.15));
#41276=CARTESIAN_POINT('Origin',(-7.5,62.5,26.15));
#41277=CARTESIAN_POINT('',(-8.625,62.5,26.225));
#41278=CARTESIAN_POINT('Origin',(-7.5,62.5,26.3));
#41279=CARTESIAN_POINT('',(-8.55,62.5,21.3));
#41280=CARTESIAN_POINT('',(-8.55,62.5,26.3));
#41281=CARTESIAN_POINT('Origin',(-7.5,62.5,21.3));
#41282=CARTESIAN_POINT('Origin',(-7.5,77.5,26.225));
#41283=CARTESIAN_POINT('',(-8.55,77.5,26.15));
#41284=CARTESIAN_POINT('Origin',(-7.5,77.5,26.15));
#41285=CARTESIAN_POINT('',(-8.625,77.5,26.225));
#41286=CARTESIAN_POINT('Origin',(-7.5,77.5,26.3));
#41287=CARTESIAN_POINT('',(-8.55,77.5,21.3));
#41288=CARTESIAN_POINT('',(-8.55,77.5,26.3));
#41289=CARTESIAN_POINT('Origin',(-7.5,77.5,21.3));
#41290=CARTESIAN_POINT('Origin',(7.5,62.5,26.225));
#41291=CARTESIAN_POINT('',(6.45,62.5,26.15));
#41292=CARTESIAN_POINT('Origin',(7.5,62.5,26.15));
#41293=CARTESIAN_POINT('',(6.375,62.5,26.225));
#41294=CARTESIAN_POINT('Origin',(7.5,62.5,26.3));
#41295=CARTESIAN_POINT('',(6.45,62.5,21.3));
#41296=CARTESIAN_POINT('',(6.45,62.5,26.3));
#41297=CARTESIAN_POINT('Origin',(7.5,62.5,21.3));
#41298=CARTESIAN_POINT('Origin',(7.5,77.5,20.9845481750105));
#41299=CARTESIAN_POINT('',(7.5,77.5,20.6690963500211));
#41300=CARTESIAN_POINT('',(6.975,77.5,20.9845481750105));
#41301=CARTESIAN_POINT('Origin',(7.5,62.5,20.9845481750105));
#41302=CARTESIAN_POINT('',(7.5,62.5,20.6690963500211));
#41303=CARTESIAN_POINT('',(6.975,62.5,20.9845481750105));
#41304=CARTESIAN_POINT('Origin',(-7.5,77.5,20.9845481750105));
#41305=CARTESIAN_POINT('',(-7.5,77.5,20.6690963500211));
#41306=CARTESIAN_POINT('',(-8.025,77.5,20.9845481750105));
#41307=CARTESIAN_POINT('Origin',(-7.5,62.5,20.9845481750105));
#41308=CARTESIAN_POINT('',(-7.5,62.5,20.6690963500211));
#41309=CARTESIAN_POINT('',(-8.025,62.5,20.9845481750105));
#41310=CARTESIAN_POINT('Origin',(0.,85.,26.15));
#41311=CARTESIAN_POINT('',(-2.05,85.,26.));
#41312=CARTESIAN_POINT('Origin',(0.,85.,26.));
#41313=CARTESIAN_POINT('',(-2.2,85.,26.15));
#41314=CARTESIAN_POINT('Origin',(0.,85.,26.3));
#41315=CARTESIAN_POINT('',(-2.05,85.,21.3));
#41316=CARTESIAN_POINT('',(-2.05,85.,26.3));
#41317=CARTESIAN_POINT('Origin',(0.,85.,21.3));
#41318=CARTESIAN_POINT('Origin',(7.5,82.5,26.15));
#41319=CARTESIAN_POINT('',(5.45,82.5,26.));
#41320=CARTESIAN_POINT('Origin',(7.5,82.5,26.));
#41321=CARTESIAN_POINT('',(5.3,82.5,26.15));
#41322=CARTESIAN_POINT('Origin',(7.5,82.5,26.3));
#41323=CARTESIAN_POINT('',(5.45,82.5,21.3));
#41324=CARTESIAN_POINT('',(5.45,82.5,26.3));
#41325=CARTESIAN_POINT('Origin',(7.5,82.5,21.3));
#41326=CARTESIAN_POINT('Origin',(7.5,57.5,26.15));
#41327=CARTESIAN_POINT('',(5.45,57.5,26.));
#41328=CARTESIAN_POINT('Origin',(7.5,57.5,26.));
#41329=CARTESIAN_POINT('',(5.3,57.5,26.15));
#41330=CARTESIAN_POINT('Origin',(7.5,57.5,26.3));
#41331=CARTESIAN_POINT('',(5.45,57.5,21.3));
#41332=CARTESIAN_POINT('',(5.45,57.5,26.3));
#41333=CARTESIAN_POINT('Origin',(7.5,57.5,21.3));
#41334=CARTESIAN_POINT('Origin',(-7.5,82.5,26.15));
#41335=CARTESIAN_POINT('',(-9.55,82.5,26.));
#41336=CARTESIAN_POINT('Origin',(-7.5,82.5,26.));
#41337=CARTESIAN_POINT('',(-9.7,82.5,26.15));
#41338=CARTESIAN_POINT('Origin',(-7.5,82.5,26.3));
#41339=CARTESIAN_POINT('',(-9.55,82.5,21.3));
#41340=CARTESIAN_POINT('',(-9.55,82.5,26.3));
#41341=CARTESIAN_POINT('Origin',(-7.5,82.5,21.3));
#41342=CARTESIAN_POINT('Origin',(-7.5,57.5,26.15));
#41343=CARTESIAN_POINT('',(-9.55,57.5,26.));
#41344=CARTESIAN_POINT('Origin',(-7.5,57.5,26.));
#41345=CARTESIAN_POINT('',(-9.7,57.5,26.15));
#41346=CARTESIAN_POINT('Origin',(-7.5,57.5,26.3));
#41347=CARTESIAN_POINT('',(-9.55,57.5,21.3));
#41348=CARTESIAN_POINT('',(-9.55,57.5,26.3));
#41349=CARTESIAN_POINT('Origin',(-7.5,57.5,21.3));
#41350=CARTESIAN_POINT('Origin',(0.,55.,26.15));
#41351=CARTESIAN_POINT('',(-2.05,55.,26.));
#41352=CARTESIAN_POINT('Origin',(0.,55.,26.));
#41353=CARTESIAN_POINT('',(-2.2,55.,26.15));
#41354=CARTESIAN_POINT('Origin',(0.,55.,26.3));
#41355=CARTESIAN_POINT('',(-2.05,55.,21.3));
#41356=CARTESIAN_POINT('',(-2.05,55.,26.3));
#41357=CARTESIAN_POINT('Origin',(0.,55.,21.3));
#41358=CARTESIAN_POINT('Origin',(0.,85.,20.6841178654968));
#41359=CARTESIAN_POINT('',(0.,85.,20.0682357309935));
#41360=CARTESIAN_POINT('',(-1.025,85.,20.6841178654968));
#41361=CARTESIAN_POINT('Origin',(0.,55.,20.6841178654968));
#41362=CARTESIAN_POINT('',(0.,55.,20.0682357309935));
#41363=CARTESIAN_POINT('',(-1.025,55.,20.6841178654968));
#41364=CARTESIAN_POINT('Origin',(7.5,82.5,20.6841178654968));
#41365=CARTESIAN_POINT('',(7.5,82.5,20.0682357309935));
#41366=CARTESIAN_POINT('',(6.475,82.5,20.6841178654968));
#41367=CARTESIAN_POINT('Origin',(7.5,57.5,20.6841178654968));
#41368=CARTESIAN_POINT('',(7.5,57.5,20.0682357309935));
#41369=CARTESIAN_POINT('',(6.475,57.5,20.6841178654968));
#41370=CARTESIAN_POINT('Origin',(-7.5,82.5,20.6841178654968));
#41371=CARTESIAN_POINT('',(-7.5,82.5,20.0682357309935));
#41372=CARTESIAN_POINT('',(-8.525,82.5,20.6841178654968));
#41373=CARTESIAN_POINT('Origin',(-7.5,57.5,20.6841178654968));
#41374=CARTESIAN_POINT('',(-7.5,57.5,20.0682357309935));
#41375=CARTESIAN_POINT('',(-8.525,57.5,20.6841178654968));
#41376=CARTESIAN_POINT('Origin',(0.,90.,13.3));
#41377=CARTESIAN_POINT('',(0.936749699759769,77.5,16.15));
#41378=CARTESIAN_POINT('',(0.936749699759769,90.,16.15));
#41379=CARTESIAN_POINT('',(0.936749699759769,90.,16.15));
#41380=CARTESIAN_POINT('',(-0.936749699759769,77.5,16.15));
#41381=CARTESIAN_POINT('Origin',(0.,77.5,13.3));
#41382=CARTESIAN_POINT('',(-0.936749699759769,90.,16.15));
#41383=CARTESIAN_POINT('',(-0.936749699759769,90.,16.15));
#41384=CARTESIAN_POINT('Origin',(0.,90.,13.3));
#41385=CARTESIAN_POINT('Origin',(0.,90.,21.225));
#41386=CARTESIAN_POINT('',(-12.5,90.,16.15));
#41387=CARTESIAN_POINT('',(-12.5,90.,16.15));
#41388=CARTESIAN_POINT('',(-12.5,90.,25.8));
#41389=CARTESIAN_POINT('',(-12.5,90.,26.3));
#41390=CARTESIAN_POINT('',(-6.25,90.,25.8));
#41391=CARTESIAN_POINT('',(-12.5,90.,16.15));
#41392=CARTESIAN_POINT('Origin',(12.5,50.,16.15));
#41393=CARTESIAN_POINT('',(-3.48245602987317,77.5,16.15));
#41394=CARTESIAN_POINT('',(6.25,77.5,16.15));
#41395=CARTESIAN_POINT('',(-7.35566243270259,77.5,16.15));
#41396=CARTESIAN_POINT('',(6.25,77.5,16.15));
#41397=CARTESIAN_POINT('',(-7.35566243270259,62.5,16.15));
#41398=CARTESIAN_POINT('',(-7.35566243270259,56.25,16.15));
#41399=CARTESIAN_POINT('',(-3.48245602987317,62.5,16.15));
#41400=CARTESIAN_POINT('',(6.25,62.5,16.15));
#41401=CARTESIAN_POINT('',(-0.936749699759769,62.5,16.15));
#41402=CARTESIAN_POINT('',(6.25,62.5,16.15));
#41403=CARTESIAN_POINT('',(-0.936749699759769,50.,16.15));
#41404=CARTESIAN_POINT('',(-0.936749699759769,50.,16.15));
#41405=CARTESIAN_POINT('',(-12.5,50.,16.15));
#41406=CARTESIAN_POINT('',(-12.5,50.,16.15));
#41407=CARTESIAN_POINT('',(-12.5,50.,16.15));
#41408=CARTESIAN_POINT('Origin',(0.,50.,13.3));
#41409=CARTESIAN_POINT('',(0.936749699759769,50.,16.15));
#41410=CARTESIAN_POINT('',(0.936749699759769,62.5,16.15));
#41411=CARTESIAN_POINT('',(0.936749699759769,50.,16.15));
#41412=CARTESIAN_POINT('Origin',(0.,50.,13.3));
#41413=CARTESIAN_POINT('Origin',(0.,62.5,13.3));
#41414=CARTESIAN_POINT('Origin',(0.,62.5,13.3));
#41415=CARTESIAN_POINT('',(3.48245602987317,62.5,16.15));
#41416=CARTESIAN_POINT('Origin',(0.,62.5,13.3));
#41417=CARTESIAN_POINT('',(6.25,62.5,16.15));
#41418=CARTESIAN_POINT('Origin',(0.,77.5,13.3));
#41419=CARTESIAN_POINT('',(3.48245602987317,77.5,16.15));
#41420=CARTESIAN_POINT('',(6.25,77.5,16.15));
#41421=CARTESIAN_POINT('Origin',(0.,77.5,13.3));
#41422=CARTESIAN_POINT('Origin',(0.,62.5,13.3));
#41423=CARTESIAN_POINT('',(-4.5,62.5,13.3));
#41424=CARTESIAN_POINT('Origin',(0.,62.5,13.3));
#41425=CARTESIAN_POINT('Origin',(0.,62.5,13.3));
#41426=CARTESIAN_POINT('',(-4.5,77.5,13.3));
#41427=CARTESIAN_POINT('',(-4.5,62.5,13.3));
#41428=CARTESIAN_POINT('Origin',(0.,77.5,13.3));
#41429=CARTESIAN_POINT('Origin',(0.,77.5,13.3));
#41430=CARTESIAN_POINT('Origin',(-6.25,50.25,26.05));
#41431=CARTESIAN_POINT('',(-12.5,50.,25.8));
#41432=CARTESIAN_POINT('',(-12.,50.5,26.3));
#41433=CARTESIAN_POINT('',(-6.25,50.,25.8));
#41434=CARTESIAN_POINT('',(12.5,50.,25.8));
#41435=CARTESIAN_POINT('Origin',(-12.25,50.,26.05));
#41436=CARTESIAN_POINT('',(-12.5,50.,25.8));
#41437=CARTESIAN_POINT('',(-12.,89.5,26.3));
#41438=CARTESIAN_POINT('Origin',(-6.25,89.75,26.05));
#41439=CARTESIAN_POINT('',(12.5,90.,25.8));
#41440=CARTESIAN_POINT('Origin',(12.25,50.,26.05));
#41441=CARTESIAN_POINT('Origin',(0.,50.,21.225));
#41442=CARTESIAN_POINT('',(-12.5,50.,16.15));
#41443=CARTESIAN_POINT('',(-12.5,50.,26.3));
#41444=CARTESIAN_POINT('Origin',(0.,77.5,12.125));
#41445=CARTESIAN_POINT('',(7.35566243270259,77.5,16.15));
#41446=CARTESIAN_POINT('',(6.25,77.5,16.15));
#41447=CARTESIAN_POINT('',(10.2135462651912,77.5,11.2));
#41448=CARTESIAN_POINT('',(10.2135462651912,77.5,11.2));
#41449=CARTESIAN_POINT('',(10.2135462651912,77.5,7.6));
#41450=CARTESIAN_POINT('',(10.2135462651912,77.5,7.6));
#41451=CARTESIAN_POINT('',(-10.2135462651912,77.5,7.6));
#41452=CARTESIAN_POINT('',(-10.2135462651912,77.5,7.6));
#41453=CARTESIAN_POINT('',(-10.2135462651912,77.5,11.2));
#41454=CARTESIAN_POINT('',(-10.2135462651912,77.5,11.2));
#41455=CARTESIAN_POINT('',(-7.35566243270259,77.5,16.15));
#41456=CARTESIAN_POINT('Origin',(-10.2135462651912,62.5,11.2));
#41457=CARTESIAN_POINT('',(-10.2135462651912,62.5,11.2));
#41458=CARTESIAN_POINT('',(-7.35566243270259,62.5,16.15));
#41459=CARTESIAN_POINT('',(-10.2135462651912,62.5,11.2));
#41460=CARTESIAN_POINT('Origin',(-10.2135462651912,62.5,7.6));
#41461=CARTESIAN_POINT('',(-10.2135462651912,62.5,7.6));
#41462=CARTESIAN_POINT('',(-10.2135462651912,62.5,11.2));
#41463=CARTESIAN_POINT('',(-10.2135462651912,62.5,7.6));
#41464=CARTESIAN_POINT('Origin',(10.2135462651912,62.5,7.6));
#41465=CARTESIAN_POINT('',(10.2135462651912,62.5,7.6));
#41466=CARTESIAN_POINT('',(-10.2135462651912,62.5,7.6));
#41467=CARTESIAN_POINT('',(10.2135462651912,62.5,7.6));
#41468=CARTESIAN_POINT('Origin',(10.2135462651912,62.5,11.2));
#41469=CARTESIAN_POINT('',(10.2135462651912,62.5,11.2));
#41470=CARTESIAN_POINT('',(10.2135462651912,62.5,7.6));
#41471=CARTESIAN_POINT('',(10.2135462651912,62.5,11.2));
#41472=CARTESIAN_POINT('Origin',(7.35566243270259,62.5,16.15));
#41473=CARTESIAN_POINT('',(7.35566243270259,62.5,16.15));
#41474=CARTESIAN_POINT('',(10.2135462651912,62.5,11.2));
#41475=CARTESIAN_POINT('',(7.35566243270259,56.25,16.15));
#41476=CARTESIAN_POINT('Origin',(0.,62.5,12.125));
#41477=CARTESIAN_POINT('',(6.25,62.5,16.15));
#41478=CARTESIAN_POINT('Origin',(-12.5,50.,16.15));
#41479=CARTESIAN_POINT('Origin',(12.5,50.,16.15));
#135255=UNCERTAINTY_MEASURE_WITH_UNIT(LENGTH_MEASURE(0.01),#135283,
'DISTANCE_ACCURACY_VALUE',
'Maximum model space distance between geometric entities at asserted c
onnectivities');
#135267=UNCERTAINTY_MEASURE_WITH_UNIT(LENGTH_MEASURE(0.01),#135283,
'DISTANCE_ACCURACY_VALUE',
'Maximum model space distance between geometric entities at asserted c
onnectivities');
#135270=(
GEOMETRIC_REPRESENTATION_CONTEXT(3)
GLOBAL_UNCERTAINTY_ASSIGNED_CONTEXT((#135255))
GLOBAL_UNIT_ASSIGNED_CONTEXT((#135283,#135285,#135286))
REPRESENTATION_CONTEXT('','3D')
);
#135282=(
GEOMETRIC_REPRESENTATION_CONTEXT(3)
GLOBAL_UNCERTAINTY_ASSIGNED_CONTEXT((#135267))
GLOBAL_UNIT_ASSIGNED_CONTEXT((#135283,#135285,#135286))
REPRESENTATION_CONTEXT('','3D')
);
#135283=(
LENGTH_UNIT()
NAMED_UNIT(*)
SI_UNIT(.MILLI.,.METRE.)
);
#135285=(
NAMED_UNIT(*)
PLANE_ANGLE_UNIT()
SI_UNIT($,.RADIAN.)
);
#135286=(
NAMED_UNIT(*)
SI_UNIT($,.STERADIAN.)
SOLID_ANGLE_UNIT()
);
#135289=SHAPE_DEFINITION_REPRESENTATION(#135303,#135338);
#135303=PRODUCT_DEFINITION_SHAPE('',$,#135353);
#135338=SHAPE_REPRESENTATION('',(#32276),#135270);
#135350=PRODUCT_DEFINITION_CONTEXT('part definition',#135394,'design');
#135353=PRODUCT_DEFINITION('2026-10-15-19-09-11-256',
'Dovetail Carriage',#135367,#135350);
#135367=PRODUCT_DEFINITION_FORMATION('',$,#135398);
#135394=APPLICATION_CONTEXT(
'Core Data for Automotive Mechanical Design Process');
#135395=PRODUCT_CONTEXT('part definition',#135394,'mechanical');
#135398=PRODUCT('2026-10-15-19-09-11-256','Dovetail Carriage',$,(#135395));
#135412=PRESENTATION_STYLE_ASSIGNMENT((#135426));
#135426=SURFACE_STYLE_USAGE(.BOTH.,#135440);
#135440=SURFACE_SIDE_STYLE('',(#135454));
#135454=SURFACE_STYLE_FILL_AREA(#135468);
#135468=FILL_AREA_STYLE('Opaque(220,223,228)',(#135482));
#135482=FILL_AREA_STYLE_COLOUR('Opaque(220,223,228)',#135496);
#135496=COLOUR_RGB('Opaque(220,223,228)', 0.66274510, 0.83137255, 0.94901961);
ENDSEC;
END-ISO-10303-21;
